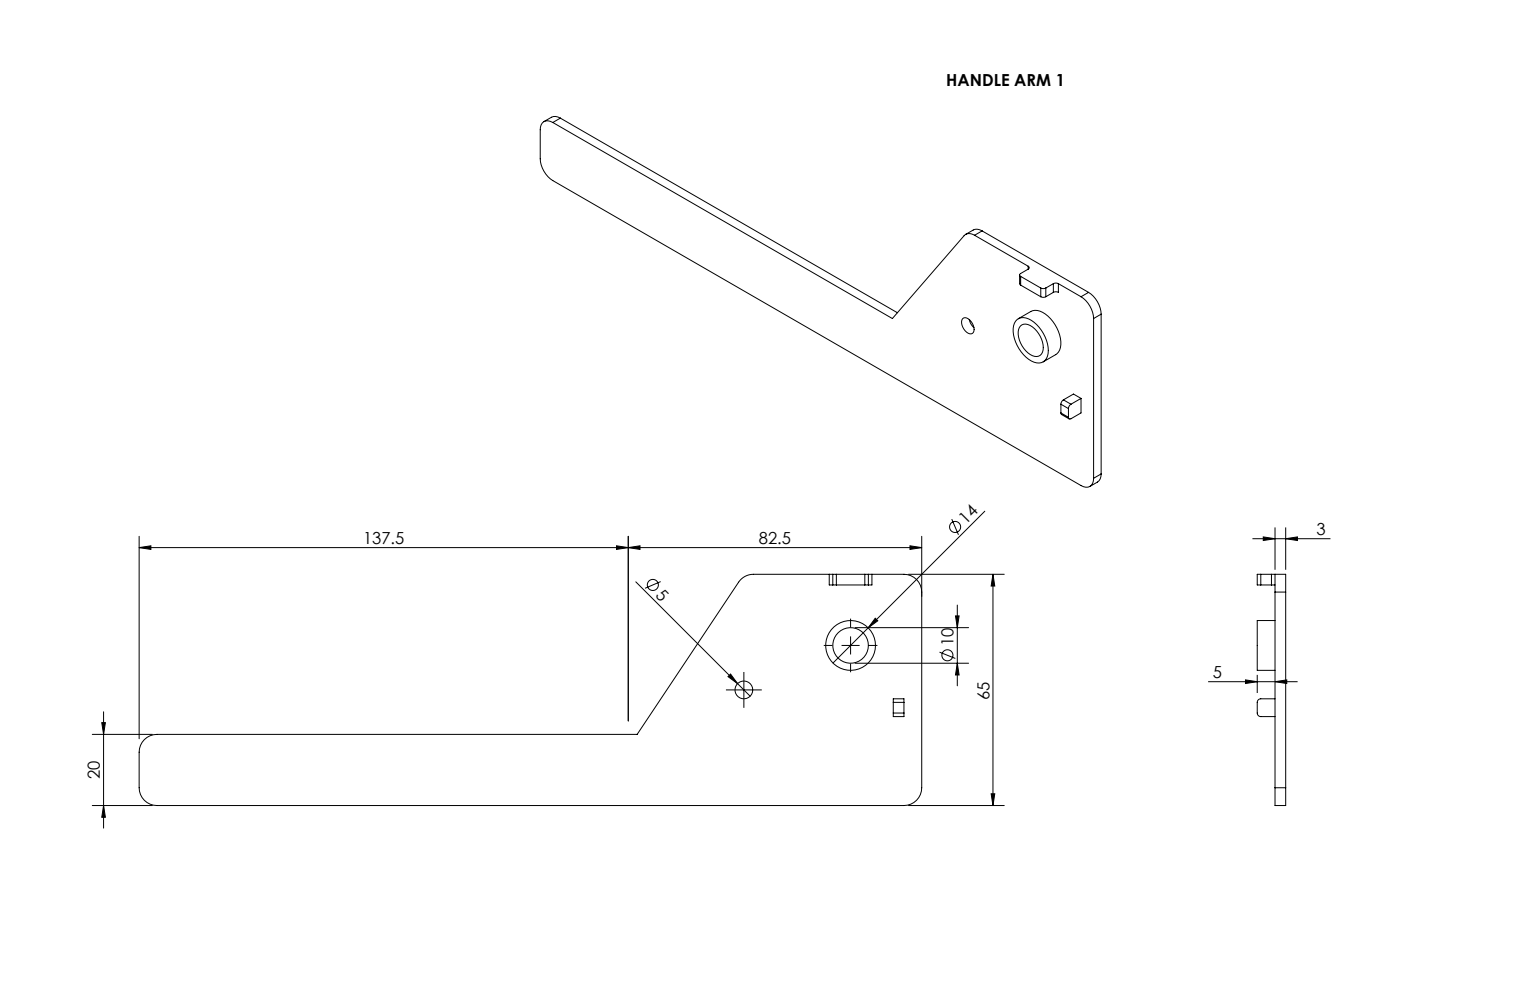
ISO-10303-21;
HEADER;
FILE_DESCRIPTION (('STEP AP214'),
    '1' );
FILE_NAME ('Handle Arm 1.step',
    '2026-09-24T10:15:42',
    ( '' ),
    ( '' ),
    'SwSTEP 2.0',
    'SolidWorks 2026',
    '' );
FILE_SCHEMA (( 'AUTOMOTIVE_DESIGN' ));
ENDSEC;

DATA;
#1=PRODUCT_DEFINITION_CONTEXT ( 'detailed design', #13776, 'design' ) ;
#12=DIRECTION ( 'NONE',  ( -1.000000000000000000, 0.000000000000000000, 0.000000000000000000 ) ) ;
#14=ORIENTED_EDGE ( 'NONE', *, *, #2662, .F. ) ;
#26=FACE_BOUND ( 'NONE', #13698, .T. ) ;
#28=DIRECTION ( 'NONE',  ( 0.000000000000000000, 0.000000000000000000, 1.000000000000000000 ) ) ;
#44=DIRECTION ( 'NONE',  ( -0.000000000000000000, 1.000000000000000000, -0.000000000000000000 ) ) ;
#93=ORIENTED_EDGE ( 'NONE', *, *, #12903, .T. ) ;
#95=CIRCLE ( 'NONE', #1308, 7.000000000000000000 ) ;
#113=ORIENTED_EDGE ( 'NONE', *, *, #10115, .F. ) ;
#155=ORIENTED_EDGE ( 'NONE', *, *, #10739, .F. ) ;
#161=AXIS2_PLACEMENT_3D ( 'NONE', #1843, #5935, #10343 ) ;
#162=CARTESIAN_POINT ( 'NONE',  ( 0.000000000000000000, 0.000000000000000000, 3.000000000000000000 ) ) ;
#198=LINE ( 'NONE', #14619, #1257 ) ;
#221=EDGE_CURVE ( 'NONE', #1746, #4825, #4915, .T. ) ;
#222=CARTESIAN_POINT ( 'NONE',  ( -199.9999999999999716, -40.00000000000003553, 0.000000000000000000 ) ) ;
#235=CARTESIAN_POINT ( 'NONE',  ( -7.000000000000000000, 0.000000000000000000, 3.000000000000000000 ) ) ;
#275=DIRECTION ( 'NONE',  ( -0.000000000000000000, -0.000000000000000000, -1.000000000000000000 ) ) ;
#276=ORIENTED_EDGE ( 'NONE', *, *, #18179, .T. ) ;
#278=ORIENTED_EDGE ( 'NONE', *, *, #5786, .T. ) ;
#313=CYLINDRICAL_SURFACE ( 'NONE', #161, 1.000000000000000000 ) ;
#317=CARTESIAN_POINT ( 'NONE',  ( 12.00000000000000711, -19.99999999999999645, 8.000000000000000000 ) ) ;
#358=AXIS2_PLACEMENT_3D ( 'NONE', #13594, #3263, #9294 ) ;
#369=VERTEX_POINT ( 'NONE', #8341 ) ;
#398=CARTESIAN_POINT ( 'NONE',  ( -59.99999999999997158, -25.00000000000000711, 3.000000000000000000 ) ) ;
#407=ORIENTED_EDGE ( 'NONE', *, *, #468, .F. ) ;
#423=ORIENTED_EDGE ( 'NONE', *, *, #6973, .T. ) ;
#425=ORIENTED_EDGE ( 'NONE', *, *, #1863, .T. ) ;
#453=CARTESIAN_POINT ( 'NONE',  ( 5.000000000000000000, 20.00000000000000000, 7.000000000000000000 ) ) ;
#460=VECTOR ( 'NONE', #9280, 1000.000000000000000 ) ;
#468=EDGE_CURVE ( 'NONE', #16237, #16692, #17037, .T. ) ;
#469=ORIENTED_EDGE ( 'NONE', *, *, #3648, .F. ) ;
#474=AXIS2_PLACEMENT_3D ( 'NONE', #15954, #2942, #11381 ) ;
#490=EDGE_CURVE ( 'NONE', #12958, #6376, #11788, .T. ) ;
#515=PLANE ( 'NONE',  #9065 ) ;
#521=ORIENTED_EDGE ( 'NONE', *, *, #6601, .T. ) ;
#522=EDGE_LOOP ( 'NONE', ( #4200, #469, #9794, #11121 ) ) ;
#530=VECTOR ( 'NONE', #4094, 1000.000000000000000 ) ;
#560=EDGE_CURVE ( 'NONE', #16555, #5753, #17707, .T. ) ;
#570=VERTEX_POINT ( 'NONE', #398 ) ;
#573=EDGE_LOOP ( 'NONE', ( #1318, #5480, #17892, #18760, #5656, #10397, #11984, #9259, #13184, #1949, #6060, #18876, #14646, #9892, #5411 ) ) ;
#585=DIRECTION ( 'NONE',  ( -0.000000000000000000, -0.000000000000000000, -1.000000000000000000 ) ) ;
#586=EDGE_CURVE ( 'NONE', #8358, #2858, #15012, .T. ) ;
#615=CARTESIAN_POINT ( 'NONE',  ( 14.99999999999999289, 20.00000000000000000, 3.000000000000000000 ) ) ;
#626=FILL_AREA_STYLE ('',( #13710 ) ) ;
#635=LINE ( 'NONE', #5205, #2069 ) ;
#648=EDGE_CURVE ( 'NONE', #1182, #5121, #7868, .T. ) ;
#692=CARTESIAN_POINT ( 'NONE',  ( 15.00000000000000711, -19.99999999999999645, 8.000000000000000000 ) ) ;
#704=ORIENTED_EDGE ( 'NONE', *, *, #13489, .F. ) ;
#745=EDGE_LOOP ( 'NONE', ( #12051, #16881, #10808, #1545 ) ) ;
#751=AXIS2_PLACEMENT_3D ( 'NONE', #1811, #13461, #4679 ) ;
#753=DIRECTION ( 'NONE',  ( -2.891205793294679312E-16, 1.000000000000000000, -0.000000000000000000 ) ) ;
#761=FACE_OUTER_BOUND ( 'NONE', #16218, .T. ) ;
#805=LINE ( 'NONE', #12460, #8156 ) ;
#815=DIRECTION ( 'NONE',  ( 0.000000000000000000, 1.000000000000000000, 0.000000000000000000 ) ) ;
#839=EDGE_LOOP ( 'NONE', ( #9618, #4136, #7135, #7088 ) ) ;
#862=LINE ( 'NONE', #2380, #530 ) ;
#864=VECTOR ( 'NONE', #14123, 1000.000000000000000 ) ;
#869=CARTESIAN_POINT ( 'NONE',  ( -31.48433267924924550, 17.77350098112614418, 3.000000000000000000 ) ) ;
#952=AXIS2_PLACEMENT_3D ( 'NONE', #17004, #15642, #4089 ) ;
#963=LINE ( 'NONE', #3481, #18162 ) ;
#964=VECTOR ( 'NONE', #10328, 1000.000000000000000 ) ;
#984=EDGE_CURVE ( 'NONE', #4000, #3723, #9255, .T. ) ;
#1011=ORIENTED_EDGE ( 'NONE', *, *, #18077, .T. ) ;
#1034=CIRCLE ( 'NONE', #6558, 5.000000000000000888 ) ;
#1077=CIRCLE ( 'NONE', #5966, 7.000000000000000000 ) ;
#1089=( GEOMETRIC_REPRESENTATION_CONTEXT ( 3 ) GLOBAL_UNCERTAINTY_ASSIGNED_CONTEXT ( ( #4604 ) ) GLOBAL_UNIT_ASSIGNED_CONTEXT ( ( #12759, #3971, #14471 ) ) REPRESENTATION_CONTEXT ( 'NONE', 'WORKASPACE' ) );
#1111=LINE ( 'NONE', #8383, #16047 ) ;
#1121=AXIS2_PLACEMENT_3D ( 'NONE', #8036, #5424, #9728 ) ;
#1130=CIRCLE ( 'NONE', #17008, 1.000000000000000000 ) ;
#1160=EDGE_CURVE ( 'NONE', #17471, #3540, #11075, .T. ) ;
#1171=UNCERTAINTY_MEASURE_WITH_UNIT (LENGTH_MEASURE( 1.000000000000000082E-05 ), #17826, 'distance_accuracy_value', 'NONE');
#1182=VERTEX_POINT ( 'NONE', #2186 ) ;
#1186=EDGE_CURVE ( 'NONE', #5607, #14673, #5331, .T. ) ;
#1194=DIRECTION ( 'NONE',  ( -0.000000000000000000, -0.000000000000000000, -1.000000000000000000 ) ) ;
#1202=( GEOMETRIC_REPRESENTATION_CONTEXT ( 3 ) GLOBAL_UNCERTAINTY_ASSIGNED_CONTEXT ( ( #1171 ) ) GLOBAL_UNIT_ASSIGNED_CONTEXT ( ( #17826, #3665, #10559 ) ) REPRESENTATION_CONTEXT ( 'NONE', 'WORKASPACE' ) );
#1221=CIRCLE ( 'NONE', #2701, 1.000000000000000000 ) ;
#1224=ADVANCED_FACE ( 'NONE', ( #6855 ), #12955, .F. ) ;
#1226=EDGE_LOOP ( 'NONE', ( #3328, #17393 ) ) ;
#1241=EDGE_CURVE ( 'NONE', #18187, #18838, #13054, .T. ) ;
#1244=DIRECTION ( 'NONE',  ( 0.000000000000000000, 0.000000000000000000, 1.000000000000000000 ) ) ;
#1257=VECTOR ( 'NONE', #4220, 1000.000000000000000 ) ;
#1308=AXIS2_PLACEMENT_3D ( 'NONE', #10783, #18228, #8012 ) ;
#1310=CARTESIAN_POINT ( 'NONE',  ( -194.9999999999999716, -25.00000000000003197, 0.000000000000000000 ) ) ;
#1318=ORIENTED_EDGE ( 'NONE', *, *, #5137, .T. ) ;
#1356=CARTESIAN_POINT ( 'NONE',  ( 0.000000000000000000, 0.000000000000000000, 3.000000000000000000 ) ) ;
#1368=DIRECTION ( 'NONE',  ( 1.000000000000000000, -0.000000000000000000, -0.000000000000000000 ) ) ;
#1385=SURFACE_SIDE_STYLE ('',( #10081 ) ) ;
#1387=LINE ( 'NONE', #17642, #18551 ) ;
#1396=COLOUR_RGB ( '', 0.66274510, 0.83137255, 0.94901961) ;
#1417=AXIS2_PLACEMENT_3D ( 'NONE', #8399, #17095, #15747 ) ;
#1429=ORIENTED_EDGE ( 'NONE', *, *, #9598, .F. ) ;
#1432=CARTESIAN_POINT ( 'NONE',  ( -199.9999999999999716, -25.00000000000003197, 3.000000000000000000 ) ) ;
#1440=CIRCLE ( 'NONE', #17939, 1.000000000000000000 ) ;
#1452=DIRECTION ( 'NONE',  ( 0.000000000000000000, 0.000000000000000000, -1.000000000000000000 ) ) ;
#1503=CARTESIAN_POINT ( 'NONE',  ( 0.000000000000000000, -15.99999999999999645, 7.000000000000000000 ) ) ;
#1544=EDGE_CURVE ( 'NONE', #14463, #9042, #14538, .T. ) ;
#1545=ORIENTED_EDGE ( 'NONE', *, *, #3989, .T. ) ;
#1566=VERTEX_POINT ( 'NONE', #9951 ) ;
#1589=FACE_OUTER_BOUND ( 'NONE', #1862, .T. ) ;
#1600=LINE ( 'NONE', #10200, #6143 ) ;
#1608=ORIENTED_EDGE ( 'NONE', *, *, #6091, .F. ) ;
#1654=VECTOR ( 'NONE', #17324, 1000.000000000000000 ) ;
#1660=ADVANCED_FACE ( 'NONE', ( #11871 ), #4607, .F. ) ;
#1668=AXIS2_PLACEMENT_3D ( 'NONE', #5688, #15832, #14585 ) ;
#1710=EDGE_CURVE ( 'NONE', #9189, #11716, #4983, .T. ) ;
#1719=( GEOMETRIC_REPRESENTATION_CONTEXT ( 3 ) GLOBAL_UNCERTAINTY_ASSIGNED_CONTEXT ( ( #13193 ) ) GLOBAL_UNIT_ASSIGNED_CONTEXT ( ( #14378, #12665, #4064 ) ) REPRESENTATION_CONTEXT ( 'NONE', 'WORKASPACE' ) );
#1721=PLANE ( 'NONE',  #4737 ) ;
#1724=ORIENTED_EDGE ( 'NONE', *, *, #586, .F. ) ;
#1743=DIRECTION ( 'NONE',  ( 1.000000000000000000, 0.000000000000000000, 0.000000000000000000 ) ) ;
#1746=VERTEX_POINT ( 'NONE', #12253 ) ;
#1751=LINE ( 'NONE', #16478, #16323 ) ;
#1759=ORIENTED_EDGE ( 'NONE', *, *, #2129, .F. ) ;
#1811=CARTESIAN_POINT ( 'NONE',  ( -194.9999999999999716, -30.00000000000003197, 3.000000000000000000 ) ) ;
#1828=ORIENTED_EDGE ( 'NONE', *, *, #2662, .T. ) ;
#1843=CARTESIAN_POINT ( 'NONE',  ( -6.000000000000000000, 20.00000000000000000, 4.000000000000000000 ) ) ;
#1862=EDGE_LOOP ( 'NONE', ( #3776, #7335, #13877, #5146 ) ) ;
#1863=EDGE_CURVE ( 'NONE', #16885, #9189, #8144, .T. ) ;
#1870=PLANE ( 'NONE',  #10860 ) ;
#1876=VECTOR ( 'NONE', #4466, 1000.000000000000000 ) ;
#1905=CARTESIAN_POINT ( 'NONE',  ( -5.000000000000000888, 17.00000000000000000, 8.000000000000000000 ) ) ;
#1909=CIRCLE ( 'NONE', #18376, 2.499999999999995115 ) ;
#1920=CARTESIAN_POINT ( 'NONE',  ( -5.000000000000000888, 17.00000000000000000, 8.000000000000000000 ) ) ;
#1949=ORIENTED_EDGE ( 'NONE', *, *, #984, .T. ) ;
#1957=FACE_OUTER_BOUND ( 'NONE', #3513, .T. ) ;
#1961=CARTESIAN_POINT ( 'NONE',  ( 12.00000000000000711, -19.99999999999999645, 3.000000000000000000 ) ) ;
#1984=VECTOR ( 'NONE', #6709, 1000.000000000000000 ) ;
#2030=AXIS2_PLACEMENT_3D ( 'NONE', #15716, #11248, #17249 ) ;
#2033=AXIS2_PLACEMENT_3D ( 'NONE', #8613, #9948, #12 ) ;
#2036=LINE ( 'NONE', #692, #12375 ) ;
#2061=AXIS2_PLACEMENT_3D ( 'NONE', #12590, #2277, #3626 ) ;
#2069=VECTOR ( 'NONE', #815, 1000.000000000000000 ) ;
#2085=CARTESIAN_POINT ( 'NONE',  ( 15.00000000000000711, -15.99999999999999645, 7.000000000000000000 ) ) ;
#2112=ADVANCED_FACE ( 'NONE', ( #18885 ), #7343, .T. ) ;
#2118=ORIENTED_EDGE ( 'NONE', *, *, #9241, .T. ) ;
#2129=EDGE_CURVE ( 'NONE', #18838, #8358, #15102, .T. ) ;
#2130=ADVANCED_FACE ( 'NONE', ( #13153 ), #17459, .T. ) ;
#2142=DIRECTION ( 'NONE',  ( 0.000000000000000000, 0.000000000000000000, -1.000000000000000000 ) ) ;
#2169=LINE ( 'NONE', #16970, #15447 ) ;
#2186=CARTESIAN_POINT ( 'NONE',  ( 5.000000000000000888, 17.00000000000000000, 4.000000000000000000 ) ) ;
#2197=CARTESIAN_POINT ( 'NONE',  ( 0.000000000000000000, 0.000000000000000000, 8.000000000000000000 ) ) ;
#2204=ADVANCED_FACE ( 'NONE', ( #17170 ), #15734, .T. ) ;
#2218=LINE ( 'NONE', #7886, #4396 ) ;
#2224=DIRECTION ( 'NONE',  ( -0.000000000000000000, 1.000000000000000000, -0.000000000000000000 ) ) ;
#2230=ORIENTED_EDGE ( 'NONE', *, *, #8585, .T. ) ;
#2231=CARTESIAN_POINT ( 'NONE',  ( 15.00000000000000711, -19.99999999999999645, 3.000000000000000000 ) ) ;
#2245=AXIS2_PLACEMENT_3D ( 'NONE', #18631, #18546, #11384 ) ;
#2254=ORIENTED_EDGE ( 'NONE', *, *, #16024, .F. ) ;
#2268=DIRECTION ( 'NONE',  ( -1.000000000000000000, -0.000000000000000000, -0.000000000000000000 ) ) ;
#2277=DIRECTION ( 'NONE',  ( 2.891205793294679312E-16, -1.000000000000000000, 0.000000000000000000 ) ) ;
#2380=CARTESIAN_POINT ( 'NONE',  ( -5.000000000000000888, 17.00000000000000000, 8.000000000000000000 ) ) ;
#2388=CARTESIAN_POINT ( 'NONE',  ( -199.9999999999999716, -30.00000000000003197, 3.000000000000000000 ) ) ;
#2390=FACE_OUTER_BOUND ( 'NONE', #11983, .T. ) ;
#2438=EDGE_LOOP ( 'NONE', ( #5584, #5199, #7981, #10841 ) ) ;
#2458=ORIENTED_EDGE ( 'NONE', *, *, #9502, .T. ) ;
#2473=LINE ( 'NONE', #5445, #8530 ) ;
#2522=CARTESIAN_POINT ( 'NONE',  ( -7.000000000000000000, 0.000000000000000000, 8.000000000000000000 ) ) ;
#2549=FACE_OUTER_BOUND ( 'NONE', #3127, .T. ) ;
#2569=ADVANCED_FACE ( 'NONE', ( #3178 ), #13135, .T. ) ;
#2604=VERTEX_POINT ( 'NONE', #13798 ) ;
#2618=DIRECTION ( 'NONE',  ( 0.000000000000000000, 0.000000000000000000, -1.000000000000000000 ) ) ;
#2635=VECTOR ( 'NONE', #275, 1000.000000000000000 ) ;
#2651=CIRCLE ( 'NONE', #16093, 5.000000000000000888 ) ;
#2662=EDGE_CURVE ( 'NONE', #15937, #17471, #13615, .T. ) ;
#2665=DIRECTION ( 'NONE',  ( 0.000000000000000000, 0.000000000000000000, -1.000000000000000000 ) ) ;
#2669=EDGE_LOOP ( 'NONE', ( #14305, #3774, #4650, #17336 ) ) ;
#2680=EDGE_CURVE ( 'NONE', #14205, #3723, #805, .T. ) ;
#2701=AXIS2_PLACEMENT_3D ( 'NONE', #16647, #16830, #5259 ) ;
#2725=DIRECTION ( 'NONE',  ( -0.000000000000000000, 0.000000000000000000, 1.000000000000000000 ) ) ;
#2732=LINE ( 'NONE', #12968, #864 ) ;
#2802=ADVANCED_FACE ( 'NONE', ( #12634 ), #18845, .F. ) ;
#2806=AXIS2_PLACEMENT_3D ( 'NONE', #2197, #12505, #6691 ) ;
#2812=DIRECTION ( 'NONE',  ( -0.000000000000000000, -0.000000000000000000, -1.000000000000000000 ) ) ;
#2824=ORIENTED_EDGE ( 'NONE', *, *, #7779, .T. ) ;
#2827=EDGE_CURVE ( 'NONE', #12087, #16455, #10055, .T. ) ;
#2850=DIRECTION ( 'NONE',  ( -0.000000000000000000, -0.000000000000000000, -1.000000000000000000 ) ) ;
#2858=VERTEX_POINT ( 'NONE', #14165 ) ;
#2878=EDGE_LOOP ( 'NONE', ( #15032, #425, #13147, #2999 ) ) ;
#2942=DIRECTION ( 'NONE',  ( 0.000000000000000000, 0.000000000000000000, 1.000000000000000000 ) ) ;
#2962=CARTESIAN_POINT ( 'NONE',  ( -31.48433267924924550, 17.77350098112614418, 3.000000000000000000 ) ) ;
#2999=ORIENTED_EDGE ( 'NONE', *, *, #18071, .F. ) ;
#3009=CARTESIAN_POINT ( 'NONE',  ( 19.99999999999999645, 20.00000000000000000, 0.000000000000000000 ) ) ;
#3045=EDGE_CURVE ( 'NONE', #9189, #8319, #3244, .T. ) ;
#3067=ORIENTED_EDGE ( 'NONE', *, *, #221, .T. ) ;
#3096=ORIENTED_EDGE ( 'NONE', *, *, #8885, .F. ) ;
#3097=ADVANCED_FACE ( 'NONE', ( #16726 ), #15371, .F. ) ;
#3101=FACE_BOUND ( 'NONE', #522, .T. ) ;
#3127=EDGE_LOOP ( 'NONE', ( #13679, #11435, #11316, #6059 ) ) ;
#3136=VERTEX_POINT ( 'NONE', #5333 ) ;
#3138=DIRECTION ( 'NONE',  ( -0.000000000000000000, -0.000000000000000000, 1.000000000000000000 ) ) ;
#3149=CARTESIAN_POINT ( 'NONE',  ( -30.00000000000000711, 20.00000000000000000, 3.000000000000000000 ) ) ;
#3167=DIRECTION ( 'NONE',  ( 1.000000000000000000, 0.000000000000000000, 0.000000000000000000 ) ) ;
#3178=FACE_OUTER_BOUND ( 'NONE', #16382, .T. ) ;
#3217=ORIENTED_EDGE ( 'NONE', *, *, #6850, .F. ) ;
#3232=DIRECTION ( 'NONE',  ( -1.000000000000000000, 0.000000000000000000, 0.000000000000000000 ) ) ;
#3244=CIRCLE ( 'NONE', #1121, 5.000000000000000888 ) ;
#3263=DIRECTION ( 'NONE',  ( 0.000000000000000000, 0.000000000000000000, -1.000000000000000000 ) ) ;
#3268=CARTESIAN_POINT ( 'NONE',  ( -5.000000000000000888, 17.00000000000000000, 3.000000000000000000 ) ) ;
#3281=AXIS2_PLACEMENT_3D ( 'NONE', #9441, #2618, #15718 ) ;
#3282=CARTESIAN_POINT ( 'NONE',  ( 12.00000000000000711, -18.99999999999999645, 7.000000000000000000 ) ) ;
#3287=CARTESIAN_POINT ( 'NONE',  ( -27.50000000000000711, -12.50000000000000178, 3.000000000000000000 ) ) ;
#3298=ORIENTED_EDGE ( 'NONE', *, *, #8499, .F. ) ;
#3328=ORIENTED_EDGE ( 'NONE', *, *, #7688, .T. ) ;
#3361=DIRECTION ( 'NONE',  ( -1.000000000000000000, 0.000000000000000000, 0.000000000000000000 ) ) ;
#3362=CARTESIAN_POINT ( 'NONE',  ( -27.32408120756002035, 15.00000000000000000, 3.000000000000000000 ) ) ;
#3368=DIRECTION ( 'NONE',  ( 2.891205793294679312E-16, -1.000000000000000000, 0.000000000000000000 ) ) ;
#3423=LINE ( 'NONE', #13460, #18761 ) ;
#3436=EDGE_CURVE ( 'NONE', #6376, #6155, #7941, .T. ) ;
#3438=EDGE_CURVE ( 'NONE', #14673, #9334, #16720, .T. ) ;
#3461=DIRECTION ( 'NONE',  ( -1.577021341797097560E-16, 1.000000000000000000, 0.000000000000000000 ) ) ;
#3462=ORIENTED_EDGE ( 'NONE', *, *, #15222, .T. ) ;
#3481=CARTESIAN_POINT ( 'NONE',  ( -59.99999999999997158, -25.00000000000000711, 3.000000000000000000 ) ) ;
#3506=AXIS2_PLACEMENT_3D ( 'NONE', #12271, #6728, #18193 ) ;
#3513=EDGE_LOOP ( 'NONE', ( #16153, #14510, #9894, #11746 ) ) ;
#3517=CIRCLE ( 'NONE', #9325, 1.000000000000000000 ) ;
#3527=ORIENTED_EDGE ( 'NONE', *, *, #15997, .T. ) ;
#3532=CYLINDRICAL_SURFACE ( 'NONE', #9933, 5.000000000000000888 ) ;
#3540=VERTEX_POINT ( 'NONE', #1961 ) ;
#3556=CARTESIAN_POINT ( 'NONE',  ( -59.99999999999997158, -25.00000000000000711, 3.000000000000000000 ) ) ;
#3557=DIRECTION ( 'NONE',  ( 0.000000000000000000, -1.000000000000000000, 0.000000000000000000 ) ) ;
#3558=FACE_OUTER_BOUND ( 'NONE', #13481, .T. ) ;
#3576=VECTOR ( 'NONE', #1452, 1000.000000000000000 ) ;
#3589=MANIFOLD_SOLID_BREP ( 'Extrude-Thin1', #12430 ) ;
#3600=ORIENTED_EDGE ( 'NONE', *, *, #15222, .F. ) ;
#3606=CYLINDRICAL_SURFACE ( 'NONE', #3281, 5.000000000000000888 ) ;
#3608=CARTESIAN_POINT ( 'NONE',  ( 4.000000000000000000, 17.00000000000000000, 8.000000000000000000 ) ) ;
#3620=CARTESIAN_POINT ( 'NONE',  ( 4.000000000000000000, 20.00000000000000000, 8.000000000000000000 ) ) ;
#3626=DIRECTION ( 'NONE',  ( 1.000000000000000000, 0.000000000000000000, 0.000000000000000000 ) ) ;
#3627=FACE_OUTER_BOUND ( 'NONE', #18651, .T. ) ;
#3648=EDGE_CURVE ( 'NONE', #3540, #11936, #5548, .T. ) ;
#3665=( NAMED_UNIT ( * ) PLANE_ANGLE_UNIT ( ) SI_UNIT ( $, .RADIAN. ) );
#3718=DIRECTION ( 'NONE',  ( -0.000000000000000000, -0.000000000000000000, 1.000000000000000000 ) ) ;
#3723=VERTEX_POINT ( 'NONE', #10050 ) ;
#3727=ADVANCED_FACE ( 'NONE', ( #5639 ), #16169, .F. ) ;
#3748=ORIENTED_EDGE ( 'NONE', *, *, #3438, .F. ) ;
#3774=ORIENTED_EDGE ( 'NONE', *, *, #468, .T. ) ;
#3776=ORIENTED_EDGE ( 'NONE', *, *, #16532, .F. ) ;
#3783=LINE ( 'NONE', #8195, #16586 ) ;
#3813=EDGE_LOOP ( 'NONE', ( #407, #14321, #14508, #13808 ) ) ;
#3844=STYLED_ITEM ( 'NONE', ( #14296 ), #10845 ) ;
#3848=ORIENTED_EDGE ( 'NONE', *, *, #6525, .F. ) ;
#3889=ORIENTED_EDGE ( 'NONE', *, *, #5137, .F. ) ;
#3960=LINE ( 'NONE', #16776, #13659 ) ;
#3971=( NAMED_UNIT ( * ) PLANE_ANGLE_UNIT ( ) SI_UNIT ( $, .RADIAN. ) );
#3989=EDGE_CURVE ( 'NONE', #369, #14405, #2473, .T. ) ;
#4000=VERTEX_POINT ( 'NONE', #2388 ) ;
#4021=DIRECTION ( 'NONE',  ( -1.000000000000000000, 0.000000000000000000, -0.000000000000000000 ) ) ;
#4064=( NAMED_UNIT ( * ) SI_UNIT ( $, .STERADIAN. ) SOLID_ANGLE_UNIT ( ) );
#4074=ADVANCED_FACE ( 'NONE', ( #17288 ), #5618, .F. ) ;
#4089=DIRECTION ( 'NONE',  ( 1.601283208593975514E-16, -1.000000000000000000, 0.000000000000000000 ) ) ;
#4094=DIRECTION ( 'NONE',  ( -0.000000000000000000, -0.000000000000000000, -1.000000000000000000 ) ) ;
#4111=DIRECTION ( 'NONE',  ( 0.000000000000000000, 0.000000000000000000, 1.000000000000000000 ) ) ;
#4119=CARTESIAN_POINT ( 'NONE',  ( 0.000000000000000000, 0.000000000000000000, 0.000000000000000000 ) ) ;
#4121=ORIENTED_EDGE ( 'NONE', *, *, #8585, .F. ) ;
#4131=DIRECTION ( 'NONE',  ( 2.891205793294679312E-16, -1.000000000000000000, 0.000000000000000000 ) ) ;
#4134=DIRECTION ( 'NONE',  ( -0.000000000000000000, -0.000000000000000000, -1.000000000000000000 ) ) ;
#4136=ORIENTED_EDGE ( 'NONE', *, *, #2680, .T. ) ;
#4164=SHAPE_REPRESENTATION_RELATIONSHIP ( 'NONE' , 'NONE' ,  #9113, #10845 ) ;
#4198=VECTOR ( 'NONE', #17813, 1000.000000000000000 ) ;
#4200=ORIENTED_EDGE ( 'NONE', *, *, #5975, .F. ) ;
#4220=DIRECTION ( 'NONE',  ( 2.891205793294679312E-16, 1.000000000000000000, -0.000000000000000000 ) ) ;
#4279=LINE ( 'NONE', #3009, #1876 ) ;
#4323=AXIS2_PLACEMENT_3D ( 'NONE', #16567, #9108, #3361 ) ;
#4374=CARTESIAN_POINT ( 'NONE',  ( 15.00000000000000711, -14.99999999999999645, 3.000000000000000000 ) ) ;
#4396=VECTOR ( 'NONE', #6434, 1000.000000000000000 ) ;
#4409=CARTESIAN_POINT ( 'NONE',  ( 5.000000000000000000, 20.00000000000000000, 8.000000000000000000 ) ) ;
#4420=CARTESIAN_POINT ( 'NONE',  ( 5.000000000000000000, 20.00000000000000000, 4.000000000000000000 ) ) ;
#4421=DIRECTION ( 'NONE',  ( 0.000000000000000000, 0.000000000000000000, -1.000000000000000000 ) ) ;
#4440=CIRCLE ( 'NONE', #9931, 1.000000000000000000 ) ;
#4451=ORIENTED_EDGE ( 'NONE', *, *, #3045, .T. ) ;
#4460=FACE_OUTER_BOUND ( 'NONE', #573, .T. ) ;
#4466=DIRECTION ( 'NONE',  ( -1.601283208593975514E-16, 1.000000000000000000, -0.000000000000000000 ) ) ;
#4471=LINE ( 'NONE', #5891, #18430 ) ;
#4482=CIRCLE ( 'NONE', #6924, 5.000000000000004441 ) ;
#4505=CARTESIAN_POINT ( 'NONE',  ( -27.32408120756002035, 20.00000000000000000, 3.000000000000000000 ) ) ;
#4509=DIRECTION ( 'NONE',  ( 1.000000000000000000, 0.000000000000000000, 0.000000000000000000 ) ) ;
#4519=DIRECTION ( 'NONE',  ( 0.000000000000000000, 0.000000000000000000, 1.000000000000000000 ) ) ;
#4587=VERTEX_POINT ( 'NONE', #453 ) ;
#4598=CYLINDRICAL_SURFACE ( 'NONE', #9372, 5.000000000000000000 ) ;
#4604=UNCERTAINTY_MEASURE_WITH_UNIT (LENGTH_MEASURE( 1.000000000000000082E-05 ), #12759, 'distance_accuracy_value', 'NONE');
#4607=PLANE ( 'NONE',  #18519 ) ;
#4612=VECTOR ( 'NONE', #7351, 1000.000000000000000 ) ;
#4626=AXIS2_PLACEMENT_3D ( 'NONE', #13967, #1244, #16931 ) ;
#4628=ORIENTED_EDGE ( 'NONE', *, *, #8885, .T. ) ;
#4650=ORIENTED_EDGE ( 'NONE', *, *, #18545, .T. ) ;
#4651=ORIENTED_EDGE ( 'NONE', *, *, #490, .F. ) ;
#4677=CARTESIAN_POINT ( 'NONE',  ( -199.9999999999999716, -25.00000000000003197, 3.000000000000000000 ) ) ;
#4679=DIRECTION ( 'NONE',  ( -1.000000000000000000, 0.000000000000000000, 0.000000000000000000 ) ) ;
#4737=AXIS2_PLACEMENT_3D ( 'NONE', #1920, #10710, #7371 ) ;
#4764=AXIS2_PLACEMENT_3D ( 'NONE', #17152, #1194, #18673 ) ;
#4788=EDGE_LOOP ( 'NONE', ( #12454, #11557 ) ) ;
#4796=DIRECTION ( 'NONE',  ( -2.891205793294679312E-16, 1.000000000000000000, 0.000000000000000000 ) ) ;
#4801=DIRECTION ( 'NONE',  ( 0.5547001962252284812, 0.8320502943378440541, 0.000000000000000000 ) ) ;
#4825=VERTEX_POINT ( 'NONE', #14330 ) ;
#4903=LINE ( 'NONE', #3556, #8350 ) ;
#4910=ORIENTED_EDGE ( 'NONE', *, *, #1863, .F. ) ;
#4915=LINE ( 'NONE', #11888, #5141 ) ;
#4942=EDGE_CURVE ( 'NONE', #18779, #4000, #5017, .T. ) ;
#4983=LINE ( 'NONE', #10819, #8456 ) ;
#5004=EDGE_CURVE ( 'NONE', #16605, #7666, #18852, .T. ) ;
#5017=CIRCLE ( 'NONE', #751, 5.000000000000004441 ) ;
#5024=EDGE_LOOP ( 'NONE', ( #18369, #18554, #12205, #13177 ) ) ;
#5058=CARTESIAN_POINT ( 'NONE',  ( -27.32408120756002035, 15.00000000000000000, 3.000000000000000000 ) ) ;
#5059=CARTESIAN_POINT ( 'NONE',  ( -7.000000000000000000, 0.000000000000000000, 8.000000000000000000 ) ) ;
#5062=AXIS2_PLACEMENT_3D ( 'NONE', #18421, #585, #5149 ) ;
#5121=VERTEX_POINT ( 'NONE', #4420 ) ;
#5135=ORIENTED_EDGE ( 'NONE', *, *, #12903, .F. ) ;
#5137=EDGE_CURVE ( 'NONE', #6376, #6854, #1751, .T. ) ;
#5141=VECTOR ( 'NONE', #13606, 1000.000000000000000 ) ;
#5146=ORIENTED_EDGE ( 'NONE', *, *, #3989, .F. ) ;
#5149=DIRECTION ( 'NONE',  ( -1.000000000000000000, 0.000000000000000000, 0.000000000000000000 ) ) ;
#5158=EDGE_CURVE ( 'NONE', #5753, #16885, #1034, .T. ) ;
#5175=FACE_OUTER_BOUND ( 'NONE', #12880, .T. ) ;
#5199=ORIENTED_EDGE ( 'NONE', *, *, #9706, .T. ) ;
#5205=CARTESIAN_POINT ( 'NONE',  ( 15.00000000000000711, -19.99999999999999645, 3.000000000000000000 ) ) ;
#5211=EDGE_CURVE ( 'NONE', #9296, #3540, #2218, .T. ) ;
#5220=CARTESIAN_POINT ( 'NONE',  ( -194.9999999999999716, -25.00000000000003197, 3.000000000000000000 ) ) ;
#5239=ADVANCED_FACE ( 'NONE', ( #3558 ), #515, .F. ) ;
#5249=ORIENTED_EDGE ( 'NONE', *, *, #648, .T. ) ;
#5259=DIRECTION ( 'NONE',  ( 0.000000000000000000, 0.000000000000000000, -1.000000000000000000 ) ) ;
#5265=CARTESIAN_POINT ( 'NONE',  ( -59.99999999999997158, -25.00000000000000711, 0.000000000000000000 ) ) ;
#5275=VERTEX_POINT ( 'NONE', #16932 ) ;
#5320=CARTESIAN_POINT ( 'NONE',  ( 12.00000000000000711, -19.99999999999999645, 8.000000000000000000 ) ) ;
#5331=CIRCLE ( 'NONE', #9601, 1.000000000000000000 ) ;
#5333=CARTESIAN_POINT ( 'NONE',  ( 12.00000000000000711, -15.99999999999999645, 8.000000000000000000 ) ) ;
#5411=ORIENTED_EDGE ( 'NONE', *, *, #490, .T. ) ;
#5412=ORIENTED_EDGE ( 'NONE', *, *, #12668, .T. ) ;
#5424=DIRECTION ( 'NONE',  ( 0.000000000000000000, 0.000000000000000000, -1.000000000000000000 ) ) ;
#5445=CARTESIAN_POINT ( 'NONE',  ( -4.000000000000000888, 17.00000000000000000, 8.000000000000000000 ) ) ;
#5448=CARTESIAN_POINT ( 'NONE',  ( 15.00000000000000711, -18.99999999999999645, 8.000000000000000000 ) ) ;
#5480=ORIENTED_EDGE ( 'NONE', *, *, #12072, .T. ) ;
#5511=ADVANCED_FACE ( 'NONE', ( #8799 ), #4598, .F. ) ;
#5548=LINE ( 'NONE', #2231, #17998 ) ;
#5564=VERTEX_POINT ( 'NONE', #7958 ) ;
#5584=ORIENTED_EDGE ( 'NONE', *, *, #7779, .F. ) ;
#5588=CARTESIAN_POINT ( 'NONE',  ( 15.00000000000000711, -45.00000000000000000, 3.000000000000000000 ) ) ;
#5607=VERTEX_POINT ( 'NONE', #12426 ) ;
#5618=PLANE ( 'NONE',  #10361 ) ;
#5637=ORIENTED_EDGE ( 'NONE', *, *, #9706, .F. ) ;
#5639=FACE_OUTER_BOUND ( 'NONE', #6609, .T. ) ;
#5656=ORIENTED_EDGE ( 'NONE', *, *, #560, .T. ) ;
#5663=CIRCLE ( 'NONE', #12999, 1.000000000000000000 ) ;
#5674=ORIENTED_EDGE ( 'NONE', *, *, #12977, .T. ) ;
#5682=CARTESIAN_POINT ( 'NONE',  ( 4.000000000000000888, 17.00000000000000000, 7.000000000000000000 ) ) ;
#5688=CARTESIAN_POINT ( 'NONE',  ( 15.00000000000000711, -39.99999999999999289, 3.000000000000000000 ) ) ;
#5699=EDGE_CURVE ( 'NONE', #11329, #12087, #13643, .T. ) ;
#5746=EDGE_CURVE ( 'NONE', #3723, #14463, #4482, .T. ) ;
#5753=VERTEX_POINT ( 'NONE', #14042 ) ;
#5779=ADVANCED_FACE ( 'NONE', ( #2549 ), #10280, .T. ) ;
#5786=EDGE_CURVE ( 'NONE', #16287, #13879, #14861, .T. ) ;
#5839=CIRCLE ( 'NONE', #15930, 5.000000000000000000 ) ;
#5844=PLANE ( 'NONE',  #15783 ) ;
#5853=AXIS2_PLACEMENT_3D ( 'NONE', #10071, #2268, #6584 ) ;
#5868=LINE ( 'NONE', #11809, #13541 ) ;
#5887=CARTESIAN_POINT ( 'NONE',  ( 5.000000000000000888, 17.00000000000000000, 8.000000000000000000 ) ) ;
#5891=CARTESIAN_POINT ( 'NONE',  ( 5.000000000000000000, 20.00000000000000000, 8.000000000000000000 ) ) ;
#5935=DIRECTION ( 'NONE',  ( 2.891205793294679312E-16, 1.000000000000000000, 0.000000000000000000 ) ) ;
#5955=CYLINDRICAL_SURFACE ( 'NONE', #6494, 2.499999999999992006 ) ;
#5966=AXIS2_PLACEMENT_3D ( 'NONE', #8128, #3718, #13940 ) ;
#5973=EDGE_CURVE ( 'NONE', #9042, #18187, #3960, .T. ) ;
#5975=EDGE_CURVE ( 'NONE', #11936, #14717, #635, .T. ) ;
#5982=ORIENTED_EDGE ( 'NONE', *, *, #3436, .T. ) ;
#5992=LINE ( 'NONE', #5887, #7683 ) ;
#6010=VECTOR ( 'NONE', #10977, 1000.000000000000000 ) ;
#6046=FACE_OUTER_BOUND ( 'NONE', #5024, .T. ) ;
#6055=ORIENTED_EDGE ( 'NONE', *, *, #6489, .F. ) ;
#6059=ORIENTED_EDGE ( 'NONE', *, *, #1544, .F. ) ;
#6060=ORIENTED_EDGE ( 'NONE', *, *, #5746, .T. ) ;
#6083=ORIENTED_EDGE ( 'NONE', *, *, #14312, .T. ) ;
#6091=EDGE_CURVE ( 'NONE', #2604, #15937, #1130, .T. ) ;
#6110=LINE ( 'NONE', #1905, #8606 ) ;
#6122=DIRECTION ( 'NONE',  ( 0.000000000000000000, 0.000000000000000000, -1.000000000000000000 ) ) ;
#6143=VECTOR ( 'NONE', #8776, 1000.000000000000000 ) ;
#6155=VERTEX_POINT ( 'NONE', #14647 ) ;
#6156=VECTOR ( 'NONE', #3557, 1000.000000000000000 ) ;
#6160=DIRECTION ( 'NONE',  ( -1.000000000000000000, 0.000000000000000000, 0.000000000000000000 ) ) ;
#6164=DIRECTION ( 'NONE',  ( 1.000000000000000000, 0.000000000000000000, -0.000000000000000000 ) ) ;
#6203=CARTESIAN_POINT ( 'NONE',  ( -27.32408120756002035, 20.00000000000000000, 0.000000000000000000 ) ) ;
#6221=CARTESIAN_POINT ( 'NONE',  ( 15.00000000000000711, -19.99999999999999645, 7.000000000000000000 ) ) ;
#6225=DIRECTION ( 'NONE',  ( 0.000000000000000000, 0.000000000000000000, 1.000000000000000000 ) ) ;
#6258=AXIS2_PLACEMENT_3D ( 'NONE', #14109, #6959, #11440 ) ;
#6262=DIRECTION ( 'NONE',  ( 0.000000000000000000, -1.000000000000000000, 0.000000000000000000 ) ) ;
#6268=AXIS2_PLACEMENT_3D ( 'NONE', #3282, #17929, #7804 ) ;
#6301=VERTEX_POINT ( 'NONE', #16572 ) ;
#6325=VECTOR ( 'NONE', #3167, 1000.000000000000000 ) ;
#6376=VERTEX_POINT ( 'NONE', #615 ) ;
#6423=ORIENTED_EDGE ( 'NONE', *, *, #15997, .F. ) ;
#6433=CYLINDRICAL_SURFACE ( 'NONE', #358, 5.000000000000000888 ) ;
#6434=DIRECTION ( 'NONE',  ( -0.000000000000000000, -1.000000000000000000, -0.000000000000000000 ) ) ;
#6442=ORIENTED_EDGE ( 'NONE', *, *, #5211, .T. ) ;
#6450=SURFACE_SIDE_STYLE ('',( #12363 ) ) ;
#6453=DIRECTION ( 'NONE',  ( -1.000000000000000000, 0.000000000000000000, -0.000000000000000000 ) ) ;
#6479=FACE_OUTER_BOUND ( 'NONE', #10978, .T. ) ;
#6489=EDGE_CURVE ( 'NONE', #4587, #5607, #9756, .T. ) ;
#6494=AXIS2_PLACEMENT_3D ( 'NONE', #17822, #9122, #8918 ) ;
#6525=EDGE_CURVE ( 'NONE', #16455, #1566, #1909, .T. ) ;
#6529=CARTESIAN_POINT ( 'NONE',  ( -199.9999999999999716, -25.00000000000003197, 0.000000000000000000 ) ) ;
#6540=PLANE ( 'NONE',  #3506 ) ;
#6558=AXIS2_PLACEMENT_3D ( 'NONE', #3362, #10254, #16086 ) ;
#6579=ORIENTED_EDGE ( 'NONE', *, *, #18312, .F. ) ;
#6584=DIRECTION ( 'NONE',  ( 0.000000000000000000, 0.000000000000000000, -1.000000000000000000 ) ) ;
#6586=LINE ( 'NONE', #7747, #11140 ) ;
#6601=EDGE_CURVE ( 'NONE', #11517, #13667, #5839, .T. ) ;
#6609=EDGE_LOOP ( 'NONE', ( #5674, #5249, #155, #17840 ) ) ;
#6636=AXIS2_PLACEMENT_3D ( 'NONE', #14126, #12696, #18527 ) ;
#6639=CIRCLE ( 'NONE', #7552, 1.000000000000000000 ) ;
#6673=ORIENTED_EDGE ( 'NONE', *, *, #9598, .T. ) ;
#6691=DIRECTION ( 'NONE',  ( -1.000000000000000000, 0.000000000000000000, 0.000000000000000000 ) ) ;
#6698=DIRECTION ( 'NONE',  ( -0.000000000000000000, -0.000000000000000000, 1.000000000000000000 ) ) ;
#6709=DIRECTION ( 'NONE',  ( 0.000000000000000000, 0.000000000000000000, -1.000000000000000000 ) ) ;
#6710=VECTOR ( 'NONE', #10899, 1000.000000000000000 ) ;
#6728=DIRECTION ( 'NONE',  ( 0.000000000000000000, -1.000000000000000000, 0.000000000000000000 ) ) ;
#6771=VECTOR ( 'NONE', #3138, 1000.000000000000000 ) ;
#6798=DIRECTION ( 'NONE',  ( -0.000000000000000000, -0.000000000000000000, -1.000000000000000000 ) ) ;
#6803=DIRECTION ( 'NONE',  ( 0.000000000000000000, 0.000000000000000000, -1.000000000000000000 ) ) ;
#6850=EDGE_CURVE ( 'NONE', #14405, #14673, #6110, .T. ) ;
#6854=VERTEX_POINT ( 'NONE', #10607 ) ;
#6855=FACE_OUTER_BOUND ( 'NONE', #18318, .T. ) ;
#6864=VECTOR ( 'NONE', #15087, 1000.000000000000000 ) ;
#6873=DIRECTION ( 'NONE',  ( 0.000000000000000000, 0.000000000000000000, -1.000000000000000000 ) ) ;
#6902=VECTOR ( 'NONE', #4796, 1000.000000000000000 ) ;
#6916=ORIENTED_EDGE ( 'NONE', *, *, #12795, .T. ) ;
#6924=AXIS2_PLACEMENT_3D ( 'NONE', #12786, #14669, #11715 ) ;
#6944=DIRECTION ( 'NONE',  ( 0.000000000000000000, 0.000000000000000000, 1.000000000000000000 ) ) ;
#6959=DIRECTION ( 'NONE',  ( -1.000000000000000000, 0.000000000000000000, 0.000000000000000000 ) ) ;
#6964=VERTEX_POINT ( 'NONE', #8118 ) ;
#6973=EDGE_CURVE ( 'NONE', #3136, #1746, #8919, .T. ) ;
#6979=LINE ( 'NONE', #15292, #8149 ) ;
#6982=ORIENTED_EDGE ( 'NONE', *, *, #12536, .T. ) ;
#6991=PLANE ( 'NONE',  #8694 ) ;
#7074=ORIENTED_EDGE ( 'NONE', *, *, #18112, .T. ) ;
#7088=ORIENTED_EDGE ( 'NONE', *, *, #8814, .T. ) ;
#7101=EDGE_LOOP ( 'NONE', ( #7074, #521 ) ) ;
#7107=CARTESIAN_POINT ( 'NONE',  ( 6.000000000000000888, 17.00000000000000000, 4.000000000000000000 ) ) ;
#7133=VERTEX_POINT ( 'NONE', #235 ) ;
#7135=ORIENTED_EDGE ( 'NONE', *, *, #984, .F. ) ;
#7159=EDGE_LOOP ( 'NONE', ( #15750, #6055, #113, #3748 ) ) ;
#7184=CARTESIAN_POINT ( 'NONE',  ( 19.99999999999999645, 15.00000000000000000, 3.000000000000000000 ) ) ;
#7200=EDGE_CURVE ( 'NONE', #7133, #16692, #18087, .T. ) ;
#7201=ADVANCED_FACE ( 'NONE', ( #13508 ), #5955, .F. ) ;
#7222=AXIS2_PLACEMENT_3D ( 'NONE', #2085, #8740, #14289 ) ;
#7235=VECTOR ( 'NONE', #6453, 1000.000000000000000 ) ;
#7241=DIRECTION ( 'NONE',  ( 2.602085213965210642E-15, 0.000000000000000000, 1.000000000000000000 ) ) ;
#7242=FACE_BOUND ( 'NONE', #13550, .T. ) ;
#7243=CYLINDRICAL_SURFACE ( 'NONE', #14834, 1.000000000000000000 ) ;
#7250=FACE_OUTER_BOUND ( 'NONE', #13130, .T. ) ;
#7272=DIRECTION ( 'NONE',  ( 1.000000000000000000, 0.000000000000000000, -0.000000000000000000 ) ) ;
#7284=ADVANCED_FACE ( 'NONE', ( #16491 ), #6540, .F. ) ;
#7289=DIRECTION ( 'NONE',  ( -0.000000000000000000, -0.000000000000000000, -1.000000000000000000 ) ) ;
#7312=ORIENTED_EDGE ( 'NONE', *, *, #2827, .T. ) ;
#7324=CARTESIAN_POINT ( 'NONE',  ( 5.000000000000000000, 6.123233995736766282E-16, 8.000000000000000000 ) ) ;
#7326=ADVANCED_FACE ( 'NONE', ( #1957 ), #7794, .F. ) ;
#7335=ORIENTED_EDGE ( 'NONE', *, *, #9135, .F. ) ;
#7341=DIRECTION ( 'NONE',  ( 2.891205793294679312E-16, 1.000000000000000000, 0.000000000000000000 ) ) ;
#7343=PLANE ( 'NONE',  #10840 ) ;
#7351=DIRECTION ( 'NONE',  ( -1.000000000000000000, 0.000000000000000000, 0.000000000000000000 ) ) ;
#7371=DIRECTION ( 'NONE',  ( 0.000000000000000000, -0.000000000000000000, 1.000000000000000000 ) ) ;
#7375=ORIENTED_EDGE ( 'NONE', *, *, #18179, .F. ) ;
#7388=CARTESIAN_POINT ( 'NONE',  ( 0.000000000000000000, 0.000000000000000000, 8.000000000000000000 ) ) ;
#7422=DIRECTION ( 'NONE',  ( 2.891205793294679312E-16, -1.000000000000000000, -0.000000000000000000 ) ) ;
#7432=PLANE ( 'NONE',  #16650 ) ;
#7458=CARTESIAN_POINT ( 'NONE',  ( -5.000000000000000000, 20.00000000000000000, 4.000000000000000000 ) ) ;
#7477=CARTESIAN_POINT ( 'NONE',  ( -30.00000000000000711, 20.00000000000000000, 3.000000000000000000 ) ) ;
#7505=DIRECTION ( 'NONE',  ( -0.000000000000000000, -0.000000000000000000, 1.000000000000000000 ) ) ;
#7552=AXIS2_PLACEMENT_3D ( 'NONE', #7107, #9593, #11323 ) ;
#7594=CARTESIAN_POINT ( 'NONE',  ( 5.000000000000000000, 6.123233995736766282E-16, 0.000000000000000000 ) ) ;
#7595=DIRECTION ( 'NONE',  ( -0.000000000000000000, -1.000000000000000000, -0.000000000000000000 ) ) ;
#7598=FACE_OUTER_BOUND ( 'NONE', #8758, .T. ) ;
#7646=CARTESIAN_POINT ( 'NONE',  ( 12.00000000000000711, -14.99999999999999645, 8.000000000000000000 ) ) ;
#7656=CARTESIAN_POINT ( 'NONE',  ( 20.00000000000000711, -39.99999999999999289, 3.000000000000000000 ) ) ;
#7666=VERTEX_POINT ( 'NONE', #7458 ) ;
#7683=VECTOR ( 'NONE', #10102, 1000.000000000000000 ) ;
#7688=EDGE_CURVE ( 'NONE', #1566, #16455, #13884, .T. ) ;
#7704=SURFACE_STYLE_USAGE ( .BOTH. , #6450 ) ;
#7747=CARTESIAN_POINT ( 'NONE',  ( 5.000000000000000000, 6.123233995736766282E-16, 3.000000000000000000 ) ) ;
#7757=FACE_OUTER_BOUND ( 'NONE', #14768, .T. ) ;
#7779=EDGE_CURVE ( 'NONE', #13879, #11517, #6586, .T. ) ;
#7791=ORIENTED_EDGE ( 'NONE', *, *, #17124, .T. ) ;
#7793=ORIENTED_EDGE ( 'NONE', *, *, #18312, .T. ) ;
#7794=PLANE ( 'NONE',  #11745 ) ;
#7804=DIRECTION ( 'NONE',  ( 0.000000000000000000, 0.000000000000000000, -1.000000000000000000 ) ) ;
#7806=EDGE_CURVE ( 'NONE', #16885, #570, #3423, .T. ) ;
#7809=CIRCLE ( 'NONE', #18459, 5.000000000000004441 ) ;
#7849=VECTOR ( 'NONE', #10561, 1000.000000000000000 ) ;
#7868=LINE ( 'NONE', #13580, #6902 ) ;
#7880=ORIENTED_EDGE ( 'NONE', *, *, #16283, .T. ) ;
#7886=CARTESIAN_POINT ( 'NONE',  ( 12.00000000000000711, -19.99999999999999645, 3.000000000000000000 ) ) ;
#7902=CARTESIAN_POINT ( 'NONE',  ( 12.00000000000000711, -14.99999999999999645, 3.000000000000000000 ) ) ;
#7917=EDGE_LOOP ( 'NONE', ( #3096, #16506, #17347, #3298 ) ) ;
#7941=LINE ( 'NONE', #12316, #6710 ) ;
#7952=COLOUR_RGB ( '', 0.66274510, 0.83137255, 0.94901961) ;
#7958=CARTESIAN_POINT ( 'NONE',  ( 6.000000000000001776, 17.00000000000000000, 3.000000000000000000 ) ) ;
#7981=ORIENTED_EDGE ( 'NONE', *, *, #15527, .T. ) ;
#7985=ORIENTED_EDGE ( 'NONE', *, *, #6091, .T. ) ;
#7988=ADVANCED_FACE ( 'NONE', ( #4460, #7242, #3101, #17260 ), #7432, .F. ) ;
#8012=DIRECTION ( 'NONE',  ( 1.000000000000000000, 0.000000000000000000, 0.000000000000000000 ) ) ;
#8036=CARTESIAN_POINT ( 'NONE',  ( -27.32408120756002035, 15.00000000000000000, 0.000000000000000000 ) ) ;
#8061=LINE ( 'NONE', #6529, #6156 ) ;
#8098=AXIS2_PLACEMENT_3D ( 'NONE', #1503, #10096, #11268 ) ;
#8118=CARTESIAN_POINT ( 'NONE',  ( -6.000000000000000888, 17.00000000000000000, 3.000000000000000000 ) ) ;
#8128=CARTESIAN_POINT ( 'NONE',  ( 0.000000000000000000, 0.000000000000000000, 3.000000000000000000 ) ) ;
#8131=MECHANICAL_DESIGN_GEOMETRIC_PRESENTATION_REPRESENTATION('',(#3844),#1719);
#8144=LINE ( 'NONE', #869, #1984 ) ;
#8149=VECTOR ( 'NONE', #6698, 1000.000000000000000 ) ;
#8156=VECTOR ( 'NONE', #16585, 1000.000000000000000 ) ;
#8195=CARTESIAN_POINT ( 'NONE',  ( -59.99999999999997158, -25.00000000000000711, 0.000000000000000000 ) ) ;
#8203=ORIENTED_EDGE ( 'NONE', *, *, #14495, .T. ) ;
#8262=CARTESIAN_POINT ( 'NONE',  ( -27.50000000000000711, -12.50000000000000178, 3.000000000000000000 ) ) ;
#8291=ORIENTED_EDGE ( 'NONE', *, *, #10957, .F. ) ;
#8297=LINE ( 'NONE', #12408, #16377 ) ;
#8317=AXIS2_PLACEMENT_3D ( 'NONE', #10456, #7505, #6160 ) ;
#8319=VERTEX_POINT ( 'NONE', #6203 ) ;
#8341=CARTESIAN_POINT ( 'NONE',  ( -4.000000000000000000, 20.00000000000000000, 8.000000000000000000 ) ) ;
#8350=VECTOR ( 'NONE', #9292, 1000.000000000000000 ) ;
#8358=VERTEX_POINT ( 'NONE', #7656 ) ;
#8369=FILL_AREA_STYLE_COLOUR ( '', #1396 ) ;
#8383=CARTESIAN_POINT ( 'NONE',  ( 12.00000000000000711, -15.99999999999999645, 8.000000000000000000 ) ) ;
#8385=ORIENTED_EDGE ( 'NONE', *, *, #17769, .T. ) ;
#8399=CARTESIAN_POINT ( 'NONE',  ( -30.00000000000000355, -12.50000000000000178, 3.000000000000000000 ) ) ;
#8417=PLANE ( 'NONE',  #2245 ) ;
#8456=VECTOR ( 'NONE', #13583, 1000.000000000000000 ) ;
#8461=DIRECTION ( 'NONE',  ( 0.000000000000000000, 1.000000000000000000, 0.000000000000000000 ) ) ;
#8481=CARTESIAN_POINT ( 'NONE',  ( -194.9999999999999716, -30.00000000000003197, 3.000000000000000000 ) ) ;
#8490=EDGE_CURVE ( 'NONE', #9334, #369, #8297, .T. ) ;
#8499=EDGE_CURVE ( 'NONE', #5275, #3136, #1111, .T. ) ;
#8530=VECTOR ( 'NONE', #12709, 1000.000000000000000 ) ;
#8538=LINE ( 'NONE', #12831, #18225 ) ;
#8566=ADVANCED_FACE ( 'NONE', ( #1589 ), #7243, .T. ) ;
#8585=EDGE_CURVE ( 'NONE', #11329, #1566, #17167, .T. ) ;
#8606=VECTOR ( 'NONE', #12033, 1000.000000000000000 ) ;
#8613=CARTESIAN_POINT ( 'NONE',  ( 14.99999999999999289, 15.00000000000000000, 3.000000000000000000 ) ) ;
#8636=EDGE_LOOP ( 'NONE', ( #278, #2824, #15357, #10482 ) ) ;
#8681=ORIENTED_EDGE ( 'NONE', *, *, #648, .F. ) ;
#8694=AXIS2_PLACEMENT_3D ( 'NONE', #18627, #10127, #2665 ) ;
#8700=LINE ( 'NONE', #4505, #964 ) ;
#8713=CARTESIAN_POINT ( 'NONE',  ( -194.9999999999999716, -45.00000000000003553, 3.000000000000000000 ) ) ;
#8740=DIRECTION ( 'NONE',  ( 1.000000000000000000, -0.000000000000000000, -0.000000000000000000 ) ) ;
#8758=EDGE_LOOP ( 'NONE', ( #9407, #14108, #6423, #13729 ) ) ;
#8772=DIRECTION ( 'NONE',  ( -1.000000000000000000, 0.000000000000000000, 0.000000000000000000 ) ) ;
#8776=DIRECTION ( 'NONE',  ( 1.000000000000000000, 1.577021341797097560E-16, -0.000000000000000000 ) ) ;
#8799=FACE_OUTER_BOUND ( 'NONE', #2438, .T. ) ;
#8802=DIRECTION ( 'NONE',  ( 1.000000000000000000, 0.000000000000000000, 0.000000000000000000 ) ) ;
#8809=EDGE_CURVE ( 'NONE', #5121, #6854, #5663, .T. ) ;
#8814=EDGE_CURVE ( 'NONE', #4000, #6301, #2169, .T. ) ;
#8851=ORIENTED_EDGE ( 'NONE', *, *, #12485, .F. ) ;
#8859=CYLINDRICAL_SURFACE ( 'NONE', #13768, 1.000000000000000000 ) ;
#8885=EDGE_CURVE ( 'NONE', #4825, #5275, #12692, .T. ) ;
#8889=ORIENTED_EDGE ( 'NONE', *, *, #10739, .T. ) ;
#8909=DIRECTION ( 'NONE',  ( 2.891205793294679312E-16, 1.000000000000000000, 0.000000000000000000 ) ) ;
#8915=ORIENTED_EDGE ( 'NONE', *, *, #1710, .F. ) ;
#8918=DIRECTION ( 'NONE',  ( -1.000000000000000000, 0.000000000000000000, 0.000000000000000000 ) ) ;
#8919=CIRCLE ( 'NONE', #5853, 1.000000000000000000 ) ;
#8928=DIRECTION ( 'NONE',  ( 0.000000000000000000, 0.000000000000000000, -1.000000000000000000 ) ) ;
#8940=ORIENTED_EDGE ( 'NONE', *, *, #12536, .F. ) ;
#8944=DIRECTION ( 'NONE',  ( 0.000000000000000000, 0.000000000000000000, -1.000000000000000000 ) ) ;
#8952=CARTESIAN_POINT ( 'NONE',  ( 19.99999999999999645, 15.00000000000000000, 3.000000000000000000 ) ) ;
#8970=CARTESIAN_POINT ( 'NONE',  ( -30.00000000000000355, -12.50000000000000178, 0.000000000000000000 ) ) ;
#8973=ORIENTED_EDGE ( 'NONE', *, *, #1241, .F. ) ;
#9012=CARTESIAN_POINT ( 'NONE',  ( 14.99999999999999289, 15.00000000000000000, 0.000000000000000000 ) ) ;
#9018=ORIENTED_EDGE ( 'NONE', *, *, #5973, .T. ) ;
#9042=VERTEX_POINT ( 'NONE', #15614 ) ;
#9065=AXIS2_PLACEMENT_3D ( 'NONE', #16656, #3461, #10833 ) ;
#9108=DIRECTION ( 'NONE',  ( 0.000000000000000000, 0.000000000000000000, -1.000000000000000000 ) ) ;
#9113=SHAPE_REPRESENTATION ( 'Handle Arm 1', ( #2030 ), #1089 ) ;
#9118=ORIENTED_EDGE ( 'NONE', *, *, #15368, .F. ) ;
#9122=DIRECTION ( 'NONE',  ( -0.000000000000000000, -0.000000000000000000, -1.000000000000000000 ) ) ;
#9135=EDGE_CURVE ( 'NONE', #17750, #16605, #14658, .T. ) ;
#9143=VECTOR ( 'NONE', #753, 1000.000000000000000 ) ;
#9180=ORIENTED_EDGE ( 'NONE', *, *, #12708, .T. ) ;
#9189=VERTEX_POINT ( 'NONE', #15324 ) ;
#9198=LINE ( 'NONE', #317, #17338 ) ;
#9202=CARTESIAN_POINT ( 'NONE',  ( -4.000000000000000888, 17.00000000000000000, 7.000000000000000000 ) ) ;
#9241=EDGE_CURVE ( 'NONE', #9042, #14205, #17245, .T. ) ;
#9255=LINE ( 'NONE', #4677, #6864 ) ;
#9259=ORIENTED_EDGE ( 'NONE', *, *, #11552, .T. ) ;
#9268=EDGE_CURVE ( 'NONE', #4825, #14717, #9411, .T. ) ;
#9280=DIRECTION ( 'NONE',  ( 0.000000000000000000, 0.000000000000000000, -1.000000000000000000 ) ) ;
#9282=ORIENTED_EDGE ( 'NONE', *, *, #18077, .F. ) ;
#9292=DIRECTION ( 'NONE',  ( -1.000000000000000000, -1.734723475976807094E-16, 0.000000000000000000 ) ) ;
#9294=DIRECTION ( 'NONE',  ( -1.000000000000000000, 0.000000000000000000, 0.000000000000000000 ) ) ;
#9296=VERTEX_POINT ( 'NONE', #7902 ) ;
#9300=FACE_OUTER_BOUND ( 'NONE', #7159, .T. ) ;
#9313=CARTESIAN_POINT ( 'NONE',  ( 7.000000000000000000, 8.572527594031473190E-16, 3.000000000000000000 ) ) ;
#9325=AXIS2_PLACEMENT_3D ( 'NONE', #18771, #8461, #6944 ) ;
#9334=VERTEX_POINT ( 'NONE', #12916 ) ;
#9353=VECTOR ( 'NONE', #7289, 1000.000000000000000 ) ;
#9372=AXIS2_PLACEMENT_3D ( 'NONE', #16158, #2850, #17491 ) ;
#9374=ORIENTED_EDGE ( 'NONE', *, *, #5158, .F. ) ;
#9398=ORIENTED_EDGE ( 'NONE', *, *, #16532, .T. ) ;
#9400=CARTESIAN_POINT ( 'NONE',  ( 4.000000000000006217, 1.156482317317873500E-15, 7.000000000000000000 ) ) ;
#9407=ORIENTED_EDGE ( 'NONE', *, *, #5004, .T. ) ;
#9411=LINE ( 'NONE', #9586, #10548 ) ;
#9441=CARTESIAN_POINT ( 'NONE',  ( 14.99999999999999289, 15.00000000000000000, 3.000000000000000000 ) ) ;
#9463=MECHANICAL_DESIGN_GEOMETRIC_PRESENTATION_REPRESENTATION('',(#17705),#1202);
#9465=ADVANCED_FACE ( 'NONE', ( #6046 ), #313, .F. ) ;
#9494=CARTESIAN_POINT ( 'NONE',  ( -59.99999999999997158, -25.00000000000000711, 3.000000000000000000 ) ) ;
#9498=DIRECTION ( 'NONE',  ( 0.000000000000000000, 0.000000000000000000, -1.000000000000000000 ) ) ;
#9501=PRODUCT_CONTEXT ( 'NONE', #12898, 'mechanical' ) ;
#9502=EDGE_CURVE ( 'NONE', #16237, #14846, #17866, .T. ) ;
#9569=FACE_BOUND ( 'NONE', #1226, .T. ) ;
#9586=CARTESIAN_POINT ( 'NONE',  ( 15.00000000000000711, -14.99999999999999645, 8.000000000000000000 ) ) ;
#9593=DIRECTION ( 'NONE',  ( 0.000000000000000000, 1.000000000000000000, 0.000000000000000000 ) ) ;
#9598=EDGE_CURVE ( 'NONE', #15937, #11936, #2036, .T. ) ;
#9601=AXIS2_PLACEMENT_3D ( 'NONE', #5682, #15629, #7241 ) ;
#9608=AXIS2_PLACEMENT_3D ( 'NONE', #7388, #4519, #1743 ) ;
#9618=ORIENTED_EDGE ( 'NONE', *, *, #12485, .T. ) ;
#9687=SHAPE_DEFINITION_REPRESENTATION ( #16065, #9113 ) ;
#9706=EDGE_CURVE ( 'NONE', #13879, #16287, #16353, .T. ) ;
#9728=DIRECTION ( 'NONE',  ( -1.000000000000000000, 0.000000000000000000, 0.000000000000000000 ) ) ;
#9739=AXIS2_PLACEMENT_3D ( 'NONE', #4409, #17313, #4131 ) ;
#9756=LINE ( 'NONE', #14258, #9808 ) ;
#9758=ADVANCED_FACE ( 'NONE', ( #2390 ), #6991, .F. ) ;
#9773=CARTESIAN_POINT ( 'NONE',  ( -5.000000000000000000, 20.00000000000000000, 8.000000000000000000 ) ) ;
#9775=DIRECTION ( 'NONE',  ( 1.000000000000000000, 1.577021341797097560E-16, -0.000000000000000000 ) ) ;
#9783=CARTESIAN_POINT ( 'NONE',  ( 6.000000000000000000, 20.00000000000000000, 4.000000000000000000 ) ) ;
#9794=ORIENTED_EDGE ( 'NONE', *, *, #5211, .F. ) ;
#9808=VECTOR ( 'NONE', #17598, 1000.000000000000000 ) ;
#9828=ORIENTED_EDGE ( 'NONE', *, *, #4942, .F. ) ;
#9852=DIRECTION ( 'NONE',  ( -1.000000000000000000, 0.000000000000000000, 0.000000000000000000 ) ) ;
#9870=VECTOR ( 'NONE', #16904, 1000.000000000000000 ) ;
#9892=ORIENTED_EDGE ( 'NONE', *, *, #15265, .T. ) ;
#9894=ORIENTED_EDGE ( 'NONE', *, *, #11552, .F. ) ;
#9903=ORIENTED_EDGE ( 'NONE', *, *, #5699, .T. ) ;
#9905=AXIS2_PLACEMENT_3D ( 'NONE', #8970, #13078, #13369 ) ;
#9911=FACE_OUTER_BOUND ( 'NONE', #10358, .T. ) ;
#9931=AXIS2_PLACEMENT_3D ( 'NONE', #10173, #44, #8928 ) ;
#9933=AXIS2_PLACEMENT_3D ( 'NONE', #5058, #18251, #10997 ) ;
#9948=DIRECTION ( 'NONE',  ( -0.000000000000000000, -0.000000000000000000, 1.000000000000000000 ) ) ;
#9951=CARTESIAN_POINT ( 'NONE',  ( -32.49999999999999289, -12.50000000000000178, 0.000000000000000000 ) ) ;
#9958=AXIS2_PLACEMENT_3D ( 'NONE', #16104, #14854, #6164 ) ;
#10000=ADVANCED_FACE ( 'NONE', ( #11427 ), #18397, .T. ) ;
#10050=CARTESIAN_POINT ( 'NONE',  ( -199.9999999999999716, -40.00000000000003553, 3.000000000000000000 ) ) ;
#10055=LINE ( 'NONE', #8262, #13016 ) ;
#10063=PLANE ( 'NONE',  #18530 ) ;
#10071=CARTESIAN_POINT ( 'NONE',  ( 12.00000000000000711, -15.99999999999999645, 7.000000000000000000 ) ) ;
#10081=SURFACE_STYLE_FILL_AREA ( #17065 ) ;
#10087=ORIENTED_EDGE ( 'NONE', *, *, #5973, .F. ) ;
#10090=ORIENTED_EDGE ( 'NONE', *, *, #5975, .T. ) ;
#10096=DIRECTION ( 'NONE',  ( 1.000000000000000000, 0.000000000000000000, 0.000000000000000000 ) ) ;
#10102=DIRECTION ( 'NONE',  ( -0.000000000000000000, -0.000000000000000000, -1.000000000000000000 ) ) ;
#10115=EDGE_CURVE ( 'NONE', #9334, #4587, #4440, .T. ) ;
#10127=DIRECTION ( 'NONE',  ( 1.000000000000000000, 0.000000000000000000, 0.000000000000000000 ) ) ;
#10135=LINE ( 'NONE', #7184, #6771 ) ;
#10173=CARTESIAN_POINT ( 'NONE',  ( 4.000000000000000000, 20.00000000000000000, 7.000000000000000000 ) ) ;
#10191=DIRECTION ( 'NONE',  ( 1.000000000000000000, 0.000000000000000000, 0.000000000000000000 ) ) ;
#10200=CARTESIAN_POINT ( 'NONE',  ( 20.00000000000000711, -45.00000000000000000, 3.000000000000000000 ) ) ;
#10254=DIRECTION ( 'NONE',  ( -0.000000000000000000, -0.000000000000000000, 1.000000000000000000 ) ) ;
#10280=CYLINDRICAL_SURFACE ( 'NONE', #17293, 5.000000000000004441 ) ;
#10288=DIRECTION ( 'NONE',  ( -1.000000000000000000, 0.000000000000000000, -0.000000000000000000 ) ) ;
#10328=DIRECTION ( 'NONE',  ( -0.000000000000000000, -0.000000000000000000, 1.000000000000000000 ) ) ;
#10343=DIRECTION ( 'NONE',  ( -1.000000000000000000, 0.000000000000000000, 0.000000000000000000 ) ) ;
#10349=CARTESIAN_POINT ( 'NONE',  ( 0.000000000000000000, 0.000000000000000000, 8.000000000000000000 ) ) ;
#10358=EDGE_LOOP ( 'NONE', ( #93, #9180, #11675, #16418 ) ) ;
#10361=AXIS2_PLACEMENT_3D ( 'NONE', #1432, #7272, #13084 ) ;
#10397=ORIENTED_EDGE ( 'NONE', *, *, #5158, .T. ) ;
#10445=DIRECTION ( 'NONE',  ( -1.000000000000000000, 0.000000000000000000, 0.000000000000000000 ) ) ;
#10454=EDGE_CURVE ( 'NONE', #14846, #7133, #11089, .T. ) ;
#10456=CARTESIAN_POINT ( 'NONE',  ( 0.000000000000000000, 0.000000000000000000, 3.000000000000000000 ) ) ;
#10477=ADVANCED_FACE ( 'NONE', ( #18252 ), #10711, .T. ) ;
#10482=ORIENTED_EDGE ( 'NONE', *, *, #15527, .F. ) ;
#10548=VECTOR ( 'NONE', #10753, 1000.000000000000000 ) ;
#10559=( NAMED_UNIT ( * ) SI_UNIT ( $, .STERADIAN. ) SOLID_ANGLE_UNIT ( ) );
#10561=DIRECTION ( 'NONE',  ( 2.891205793294679312E-16, 1.000000000000000000, -0.000000000000000000 ) ) ;
#10588=CARTESIAN_POINT ( 'NONE',  ( 12.00000000000000711, -19.99999999999999645, 7.000000000000000000 ) ) ;
#10607=CARTESIAN_POINT ( 'NONE',  ( 5.999999999999998224, 20.00000000000000000, 3.000000000000000000 ) ) ;
#10648=VERTEX_POINT ( 'NONE', #1310 ) ;
#10691=CARTESIAN_POINT ( 'NONE',  ( 15.00000000000000711, -45.00000000000000000, 3.000000000000000000 ) ) ;
#10710=DIRECTION ( 'NONE',  ( 0.000000000000000000, 1.000000000000000000, 0.000000000000000000 ) ) ;
#10711=CYLINDRICAL_SURFACE ( 'NONE', #2806, 7.000000000000000000 ) ;
#10735=FACE_OUTER_BOUND ( 'NONE', #13191, .T. ) ;
#10739=EDGE_CURVE ( 'NONE', #4587, #5121, #4471, .T. ) ;
#10745=ORIENTED_EDGE ( 'NONE', *, *, #8499, .T. ) ;
#10753=DIRECTION ( 'NONE',  ( -0.000000000000000000, -0.000000000000000000, -1.000000000000000000 ) ) ;
#10755=PRODUCT ( 'Handle Arm 1', 'Handle Arm 1', '', ( #9501 ) ) ;
#10783=CARTESIAN_POINT ( 'NONE',  ( 0.000000000000000000, 0.000000000000000000, 8.000000000000000000 ) ) ;
#10808=ORIENTED_EDGE ( 'NONE', *, *, #8490, .T. ) ;
#10819=CARTESIAN_POINT ( 'NONE',  ( -30.00000000000000711, 20.00000000000000000, 0.000000000000000000 ) ) ;
#10831=EDGE_CURVE ( 'NONE', #14846, #16237, #95, .T. ) ;
#10833=DIRECTION ( 'NONE',  ( -1.000000000000000000, -1.577021341797097560E-16, 0.000000000000000000 ) ) ;
#10840=AXIS2_PLACEMENT_3D ( 'NONE', #15925, #2725, #10191 ) ;
#10841=ORIENTED_EDGE ( 'NONE', *, *, #6601, .F. ) ;
#10845=ADVANCED_BREP_SHAPE_REPRESENTATION ( '', ( #3589, #2030 ), #1089 ) ;
#10860=AXIS2_PLACEMENT_3D ( 'NONE', #12614, #6262, #14059 ) ;
#10888=VECTOR ( 'NONE', #2812, 1000.000000000000000 ) ;
#10899=DIRECTION ( 'NONE',  ( 0.000000000000000000, 0.000000000000000000, -1.000000000000000000 ) ) ;
#10949=CARTESIAN_POINT ( 'NONE',  ( 12.00000000000000711, -19.99999999999999645, 7.000000000000000000 ) ) ;
#10957=EDGE_CURVE ( 'NONE', #11716, #10648, #3783, .T. ) ;
#10977=DIRECTION ( 'NONE',  ( -2.891205793294679312E-16, -1.000000000000000000, 0.000000000000000000 ) ) ;
#10978=EDGE_LOOP ( 'NONE', ( #4651, #17317, #9118, #14284 ) ) ;
#10981=ORIENTED_EDGE ( 'NONE', *, *, #2827, .F. ) ;
#10997=DIRECTION ( 'NONE',  ( -1.000000000000000000, 0.000000000000000000, 0.000000000000000000 ) ) ;
#11026=CARTESIAN_POINT ( 'NONE',  ( -27.50000000000000711, -12.50000000000000178, 0.000000000000000000 ) ) ;
#11028=ORIENTED_EDGE ( 'NONE', *, *, #8809, .F. ) ;
#11031=DIRECTION ( 'NONE',  ( 1.000000000000000000, 1.734723475976806848E-16, 0.000000000000000000 ) ) ;
#11075=LINE ( 'NONE', #5320, #17859 ) ;
#11089=LINE ( 'NONE', #5059, #9870 ) ;
#11121=ORIENTED_EDGE ( 'NONE', *, *, #13472, .F. ) ;
#11140=VECTOR ( 'NONE', #12139, 1000.000000000000000 ) ;
#11145=DIRECTION ( 'NONE',  ( 0.000000000000000000, -1.000000000000000000, 0.000000000000000000 ) ) ;
#11248=DIRECTION ( 'NONE',  ( 0.000000000000000000, 0.000000000000000000, 1.000000000000000000 ) ) ;
#11268=DIRECTION ( 'NONE',  ( 0.000000000000000000, 0.000000000000000000, -1.000000000000000000 ) ) ;
#11294=DIRECTION ( 'NONE',  ( 1.000000000000000000, 0.000000000000000000, -0.000000000000000000 ) ) ;
#11316=ORIENTED_EDGE ( 'NONE', *, *, #9241, .F. ) ;
#11323=DIRECTION ( 'NONE',  ( 0.000000000000000000, 0.000000000000000000, 1.000000000000000000 ) ) ;
#11329=VERTEX_POINT ( 'NONE', #15602 ) ;
#11381=DIRECTION ( 'NONE',  ( 1.000000000000000000, 0.000000000000000000, 0.000000000000000000 ) ) ;
#11384=DIRECTION ( 'NONE',  ( 0.000000000000000000, 0.000000000000000000, 1.000000000000000000 ) ) ;
#11427=FACE_OUTER_BOUND ( 'NONE', #3813, .T. ) ;
#11435=ORIENTED_EDGE ( 'NONE', *, *, #2680, .F. ) ;
#11440=DIRECTION ( 'NONE',  ( 0.000000000000000000, 0.000000000000000000, 1.000000000000000000 ) ) ;
#11514=ORIENTED_EDGE ( 'NONE', *, *, #3045, .F. ) ;
#11517=VERTEX_POINT ( 'NONE', #7594 ) ;
#11549=PLANE ( 'NONE',  #952 ) ;
#11552=EDGE_CURVE ( 'NONE', #570, #18779, #4903, .T. ) ;
#11557=ORIENTED_EDGE ( 'NONE', *, *, #18545, .F. ) ;
#11634=PRODUCT_DEFINITION ( 'UNKNOWN', '', #12039, #1 ) ;
#11675=ORIENTED_EDGE ( 'NONE', *, *, #15265, .F. ) ;
#11691=ADVANCED_FACE ( 'NONE', ( #5175 ), #8417, .F. ) ;
#11715=DIRECTION ( 'NONE',  ( -1.000000000000000000, 0.000000000000000000, 0.000000000000000000 ) ) ;
#11716=VERTEX_POINT ( 'NONE', #5265 ) ;
#11745=AXIS2_PLACEMENT_3D ( 'NONE', #9494, #12184, #11031 ) ;
#11746=ORIENTED_EDGE ( 'NONE', *, *, #18071, .T. ) ;
#11768=CARTESIAN_POINT ( 'NONE',  ( 0.000000000000000000, 0.000000000000000000, 0.000000000000000000 ) ) ;
#11788=CIRCLE ( 'NONE', #2033, 5.000000000000000888 ) ;
#11794=ORIENTED_EDGE ( 'NONE', *, *, #8814, .F. ) ;
#11809=CARTESIAN_POINT ( 'NONE',  ( 6.000000000000000888, 17.00000000000000000, 3.000000000000000000 ) ) ;
#11871=FACE_OUTER_BOUND ( 'NONE', #2878, .T. ) ;
#11882=FACE_OUTER_BOUND ( 'NONE', #18623, .T. ) ;
#11888=CARTESIAN_POINT ( 'NONE',  ( 15.00000000000000711, -14.99999999999999645, 7.000000000000000000 ) ) ;
#11911=ORIENTED_EDGE ( 'NONE', *, *, #9268, .F. ) ;
#11936=VERTEX_POINT ( 'NONE', #17786 ) ;
#11961=DIRECTION ( 'NONE',  ( -1.000000000000000000, -0.000000000000000000, -0.000000000000000000 ) ) ;
#11983=EDGE_LOOP ( 'NONE', ( #17492, #1011, #16615, #423, #15354, #6442 ) ) ;
#11984=ORIENTED_EDGE ( 'NONE', *, *, #7806, .T. ) ;
#12033=DIRECTION ( 'NONE',  ( 1.000000000000000000, 0.000000000000000000, 0.000000000000000000 ) ) ;
#12039=PRODUCT_DEFINITION_FORMATION_WITH_SPECIFIED_SOURCE ( 'ANY', '', #10755, .NOT_KNOWN. ) ;
#12051=ORIENTED_EDGE ( 'NONE', *, *, #6850, .T. ) ;
#12065=AXIS2_PLACEMENT_3D ( 'NONE', #17200, #4111, #12611 ) ;
#12072=EDGE_CURVE ( 'NONE', #6854, #5564, #5868, .T. ) ;
#12078=CARTESIAN_POINT ( 'NONE',  ( -5.000000000000000000, 0.000000000000000000, 3.000000000000000000 ) ) ;
#12080=ORIENTED_EDGE ( 'NONE', *, *, #14495, .F. ) ;
#12087=VERTEX_POINT ( 'NONE', #3287 ) ;
#12139=DIRECTION ( 'NONE',  ( -0.000000000000000000, -0.000000000000000000, -1.000000000000000000 ) ) ;
#12184=DIRECTION ( 'NONE',  ( 1.734723475976806848E-16, -1.000000000000000000, 0.000000000000000000 ) ) ;
#12205=ORIENTED_EDGE ( 'NONE', *, *, #17769, .F. ) ;
#12252=VERTEX_POINT ( 'NONE', #18384 ) ;
#12253=CARTESIAN_POINT ( 'NONE',  ( 12.00000000000000711, -14.99999999999999645, 7.000000000000000000 ) ) ;
#12267=ORIENTED_EDGE ( 'NONE', *, *, #560, .F. ) ;
#12271=CARTESIAN_POINT ( 'NONE',  ( 15.00000000000000711, -14.99999999999999645, 8.000000000000000000 ) ) ;
#12316=CARTESIAN_POINT ( 'NONE',  ( 14.99999999999999289, 20.00000000000000000, 3.000000000000000000 ) ) ;
#12363=SURFACE_STYLE_FILL_AREA ( #626 ) ;
#12375=VECTOR ( 'NONE', #12522, 1000.000000000000000 ) ;
#12395=LINE ( 'NONE', #18230, #6010 ) ;
#12408=CARTESIAN_POINT ( 'NONE',  ( -5.000000000000000000, 20.00000000000000000, 8.000000000000000000 ) ) ;
#12426=CARTESIAN_POINT ( 'NONE',  ( 5.000000000000000888, 17.00000000000000000, 7.000000000000000000 ) ) ;
#12430=CLOSED_SHELL ( 'NONE', ( #10477, #18464, #2802, #7988, #12612, #1660, #7326, #4074, #5239, #13336, #18009, #5511, #7201, #5779, #2204, #18531, #13703, #12512, #1224, #7284, #9758, #11691, #2569, #15362, #18289, #3727, #2112, #13035, #2130, #3097, #9465, #16503, #8566, #10000, #15427 ) ) ;
#12454=ORIENTED_EDGE ( 'NONE', *, *, #7200, .F. ) ;
#12460=CARTESIAN_POINT ( 'NONE',  ( -199.9999999999999716, -40.00000000000003553, 3.000000000000000000 ) ) ;
#12485=EDGE_CURVE ( 'NONE', #6301, #14205, #8061, .T. ) ;
#12505=DIRECTION ( 'NONE',  ( -0.000000000000000000, -0.000000000000000000, -1.000000000000000000 ) ) ;
#12509=CARTESIAN_POINT ( 'NONE',  ( -194.9999999999999716, -40.00000000000003553, 3.000000000000000000 ) ) ;
#12512=ADVANCED_FACE ( 'NONE', ( #10735 ), #6433, .T. ) ;
#12522=DIRECTION ( 'NONE',  ( -0.000000000000000000, -0.000000000000000000, -1.000000000000000000 ) ) ;
#12536=EDGE_CURVE ( 'NONE', #2858, #18187, #16221, .T. ) ;
#12590=CARTESIAN_POINT ( 'NONE',  ( 6.000000000000000000, 20.00000000000000000, 4.000000000000000000 ) ) ;
#12611=DIRECTION ( 'NONE',  ( 1.000000000000000000, 0.000000000000000000, 0.000000000000000000 ) ) ;
#12612=ADVANCED_FACE ( 'NONE', ( #17030, #9569, #18362 ), #17205, .T. ) ;
#12614=CARTESIAN_POINT ( 'NONE',  ( -30.00000000000000711, 20.00000000000000000, 3.000000000000000000 ) ) ;
#12634=FACE_OUTER_BOUND ( 'NONE', #8636, .T. ) ;
#12647=DIRECTION ( 'NONE',  ( -1.601283208593975514E-16, 1.000000000000000000, -0.000000000000000000 ) ) ;
#12663=CIRCLE ( 'NONE', #474, 5.000000000000000000 ) ;
#12665=( NAMED_UNIT ( * ) PLANE_ANGLE_UNIT ( ) SI_UNIT ( $, .RADIAN. ) );
#12668=EDGE_CURVE ( 'NONE', #12087, #11329, #15303, .T. ) ;
#12692=CIRCLE ( 'NONE', #7222, 1.000000000000000000 ) ;
#12696=DIRECTION ( 'NONE',  ( 0.000000000000000000, 0.000000000000000000, 1.000000000000000000 ) ) ;
#12708=EDGE_CURVE ( 'NONE', #14346, #12958, #10135, .T. ) ;
#12709=DIRECTION ( 'NONE',  ( -2.891205793294679312E-16, -1.000000000000000000, 0.000000000000000000 ) ) ;
#12749=EDGE_CURVE ( 'NONE', #6964, #16555, #198, .T. ) ;
#12759=( LENGTH_UNIT ( ) NAMED_UNIT ( * ) SI_UNIT ( .MILLI., .METRE. ) );
#12786=CARTESIAN_POINT ( 'NONE',  ( -194.9999999999999716, -40.00000000000003553, 3.000000000000000000 ) ) ;
#12795=EDGE_CURVE ( 'NONE', #8319, #5753, #8700, .T. ) ;
#12831=CARTESIAN_POINT ( 'NONE',  ( 19.99999999999999645, 20.00000000000000000, 3.000000000000000000 ) ) ;
#12865=DIRECTION ( 'NONE',  ( -1.000000000000000000, 0.000000000000000000, 0.000000000000000000 ) ) ;
#12880=EDGE_LOOP ( 'NONE', ( #1429, #1828, #16159, #14850 ) ) ;
#12897=CARTESIAN_POINT ( 'NONE',  ( 15.00000000000000711, -45.00000000000000000, 0.000000000000000000 ) ) ;
#12898=APPLICATION_CONTEXT ( 'automotive_design' ) ;
#12903=EDGE_CURVE ( 'NONE', #2858, #14346, #4279, .T. ) ;
#12916=CARTESIAN_POINT ( 'NONE',  ( 4.000000000000000888, 20.00000000000000000, 8.000000000000000000 ) ) ;
#12955=PLANE ( 'NONE',  #6258 ) ;
#12956=CIRCLE ( 'NONE', #6268, 1.000000000000000000 ) ;
#12958=VERTEX_POINT ( 'NONE', #8952 ) ;
#12968=CARTESIAN_POINT ( 'NONE',  ( 15.00000000000000711, -19.99999999999999645, 8.000000000000000000 ) ) ;
#12977=EDGE_CURVE ( 'NONE', #5607, #1182, #5992, .T. ) ;
#12999=AXIS2_PLACEMENT_3D ( 'NONE', #9783, #11145, #14006 ) ;
#13016=VECTOR ( 'NONE', #4134, 1000.000000000000000 ) ;
#13025=CARTESIAN_POINT ( 'NONE',  ( 15.00000000000000711, -18.99999999999999645, 7.000000000000000000 ) ) ;
#13035=ADVANCED_FACE ( 'NONE', ( #7250 ), #8859, .T. ) ;
#13043=DIRECTION ( 'NONE',  ( -1.000000000000000000, -0.000000000000000000, -0.000000000000000000 ) ) ;
#13049=ORIENTED_EDGE ( 'NONE', *, *, #5699, .F. ) ;
#13054=LINE ( 'NONE', #5588, #16930 ) ;
#13056=DIRECTION ( 'NONE',  ( -1.000000000000000000, 2.891205793294679805E-16, 0.000000000000000000 ) ) ;
#13061=DIRECTION ( 'NONE',  ( 0.000000000000000000, 0.000000000000000000, 1.000000000000000000 ) ) ;
#13078=DIRECTION ( 'NONE',  ( 0.000000000000000000, 0.000000000000000000, 1.000000000000000000 ) ) ;
#13084=DIRECTION ( 'NONE',  ( -0.000000000000000000, 0.000000000000000000, -1.000000000000000000 ) ) ;
#13103=DIRECTION ( 'NONE',  ( 0.000000000000000000, 0.000000000000000000, 1.000000000000000000 ) ) ;
#13130=EDGE_LOOP ( 'NONE', ( #9282, #14, #1608, #7375 ) ) ;
#13135=PLANE ( 'NONE',  #9958 ) ;
#13147=ORIENTED_EDGE ( 'NONE', *, *, #1710, .T. ) ;
#13153=FACE_OUTER_BOUND ( 'NONE', #7917, .T. ) ;
#13177=ORIENTED_EDGE ( 'NONE', *, *, #14767, .F. ) ;
#13184=ORIENTED_EDGE ( 'NONE', *, *, #4942, .T. ) ;
#13191=EDGE_LOOP ( 'NONE', ( #1759, #8973, #8940, #1724 ) ) ;
#13193=UNCERTAINTY_MEASURE_WITH_UNIT (LENGTH_MEASURE( 1.000000000000000082E-05 ), #14378, 'distance_accuracy_value', 'NONE');
#13312=CARTESIAN_POINT ( 'NONE',  ( -5.000000000000000000, 0.000000000000000000, 8.000000000000000000 ) ) ;
#13336=ADVANCED_FACE ( 'NONE', ( #9911 ), #11549, .F. ) ;
#13354=CARTESIAN_POINT ( 'NONE',  ( 0.000000000000000000, -18.99999999999999645, 7.000000000000000000 ) ) ;
#13359=LINE ( 'NONE', #7646, #2635 ) ;
#13361=VERTEX_POINT ( 'NONE', #14039 ) ;
#13369=DIRECTION ( 'NONE',  ( 1.000000000000000000, 0.000000000000000000, 0.000000000000000000 ) ) ;
#13403=DIRECTION ( 'NONE',  ( -1.000000000000000000, -0.000000000000000000, -0.000000000000000000 ) ) ;
#13460=CARTESIAN_POINT ( 'NONE',  ( -30.00000000000000711, 20.00000000000000000, 3.000000000000000000 ) ) ;
#13461=DIRECTION ( 'NONE',  ( -0.000000000000000000, -0.000000000000000000, 1.000000000000000000 ) ) ;
#13472=EDGE_CURVE ( 'NONE', #14717, #9296, #16029, .T. ) ;
#13481=EDGE_LOOP ( 'NONE', ( #704, #15408, #9018, #17721 ) ) ;
#13489=EDGE_CURVE ( 'NONE', #14463, #18838, #1600, .T. ) ;
#13508=FACE_OUTER_BOUND ( 'NONE', #14460, .T. ) ;
#13541=VECTOR ( 'NONE', #7422, 1000.000000000000000 ) ;
#13550=EDGE_LOOP ( 'NONE', ( #13049, #16315 ) ) ;
#13580=CARTESIAN_POINT ( 'NONE',  ( 5.000000000000000000, 20.00000000000000000, 4.000000000000000000 ) ) ;
#13583=DIRECTION ( 'NONE',  ( -0.5547001962252284812, -0.8320502943378440541, 0.000000000000000000 ) ) ;
#13594=CARTESIAN_POINT ( 'NONE',  ( 15.00000000000000711, -39.99999999999999289, 3.000000000000000000 ) ) ;
#13606=DIRECTION ( 'NONE',  ( 1.000000000000000000, -0.000000000000000000, -0.000000000000000000 ) ) ;
#13615=LINE ( 'NONE', #10949, #7235 ) ;
#13643=CIRCLE ( 'NONE', #1417, 2.499999999999995115 ) ;
#13658=ORIENTED_EDGE ( 'NONE', *, *, #7688, .F. ) ;
#13659=VECTOR ( 'NONE', #9775, 1000.000000000000000 ) ;
#13662=AXIS2_PLACEMENT_3D ( 'NONE', #9202, #16658, #18003 ) ;
#13667=VERTEX_POINT ( 'NONE', #16704 ) ;
#13679=ORIENTED_EDGE ( 'NONE', *, *, #5746, .F. ) ;
#13698=EDGE_LOOP ( 'NONE', ( #16596, #5637 ) ) ;
#13703=ADVANCED_FACE ( 'NONE', ( #6479 ), #3606, .T. ) ;
#13710=FILL_AREA_STYLE_COLOUR ( '', #7952 ) ;
#13729=ORIENTED_EDGE ( 'NONE', *, *, #9135, .T. ) ;
#13768=AXIS2_PLACEMENT_3D ( 'NONE', #13354, #8772, #13061 ) ;
#13776=APPLICATION_CONTEXT ( 'automotive_design' ) ;
#13787=CARTESIAN_POINT ( 'NONE',  ( -4.000000000000000000, 20.00000000000000000, 7.000000000000000000 ) ) ;
#13798=CARTESIAN_POINT ( 'NONE',  ( 15.00000000000000711, -18.99999999999999645, 8.000000000000000000 ) ) ;
#13808=ORIENTED_EDGE ( 'NONE', *, *, #7200, .T. ) ;
#13877=ORIENTED_EDGE ( 'NONE', *, *, #15551, .F. ) ;
#13878=AXIS2_PLACEMENT_3D ( 'NONE', #8481, #14310, #12865 ) ;
#13879=VERTEX_POINT ( 'NONE', #7324 ) ;
#13884=CIRCLE ( 'NONE', #9905, 2.499999999999995115 ) ;
#13893=EDGE_CURVE ( 'NONE', #6155, #8319, #1387, .T. ) ;
#13940=DIRECTION ( 'NONE',  ( -1.000000000000000000, 0.000000000000000000, 0.000000000000000000 ) ) ;
#13953=ORIENTED_EDGE ( 'NONE', *, *, #9268, .T. ) ;
#13967=CARTESIAN_POINT ( 'NONE',  ( -30.00000000000000355, -12.50000000000000178, 3.000000000000000000 ) ) ;
#14006=DIRECTION ( 'NONE',  ( 0.000000000000000000, 0.000000000000000000, -1.000000000000000000 ) ) ;
#14036=CYLINDRICAL_SURFACE ( 'NONE', #5062, 2.499999999999992006 ) ;
#14039=CARTESIAN_POINT ( 'NONE',  ( 12.00000000000000711, -18.99999999999999645, 8.000000000000000000 ) ) ;
#14042=CARTESIAN_POINT ( 'NONE',  ( -27.32408120756002035, 20.00000000000000000, 3.000000000000000000 ) ) ;
#14059=DIRECTION ( 'NONE',  ( 0.000000000000000000, -0.000000000000000000, -1.000000000000000000 ) ) ;
#14079=DIRECTION ( 'NONE',  ( -1.000000000000000000, 0.000000000000000000, 0.000000000000000000 ) ) ;
#14108=ORIENTED_EDGE ( 'NONE', *, *, #14767, .T. ) ;
#14109=CARTESIAN_POINT ( 'NONE',  ( 15.00000000000000711, -19.99999999999999645, 8.000000000000000000 ) ) ;
#14111=DIRECTION ( 'NONE',  ( -1.000000000000000000, -0.000000000000000000, -0.000000000000000000 ) ) ;
#14123=DIRECTION ( 'NONE',  ( 0.000000000000000000, 1.000000000000000000, 0.000000000000000000 ) ) ;
#14126=CARTESIAN_POINT ( 'NONE',  ( 0.000000000000000000, 0.000000000000000000, 8.000000000000000000 ) ) ;
#14165=CARTESIAN_POINT ( 'NONE',  ( 20.00000000000000711, -39.99999999999999289, 0.000000000000000000 ) ) ;
#14205=VERTEX_POINT ( 'NONE', #222 ) ;
#14228=DIRECTION ( 'NONE',  ( -1.000000000000000000, 0.000000000000000000, 0.000000000000000000 ) ) ;
#14255=EDGE_LOOP ( 'NONE', ( #9828, #2254, #6579, #11794 ) ) ;
#14258=CARTESIAN_POINT ( 'NONE',  ( 5.000000000000000888, 17.00000000000000000, 7.000000000000000000 ) ) ;
#14271=DIRECTION ( 'NONE',  ( -0.000000000000000000, -0.000000000000000000, -1.000000000000000000 ) ) ;
#14284=ORIENTED_EDGE ( 'NONE', *, *, #3436, .F. ) ;
#14289=DIRECTION ( 'NONE',  ( 0.000000000000000000, 0.000000000000000000, 1.000000000000000000 ) ) ;
#14296=PRESENTATION_STYLE_ASSIGNMENT (( #15814 ) ) ;
#14305=ORIENTED_EDGE ( 'NONE', *, *, #9502, .F. ) ;
#14310=DIRECTION ( 'NONE',  ( 0.000000000000000000, 0.000000000000000000, -1.000000000000000000 ) ) ;
#14312=EDGE_CURVE ( 'NONE', #3136, #13361, #9198, .T. ) ;
#14321=ORIENTED_EDGE ( 'NONE', *, *, #10831, .F. ) ;
#14330=CARTESIAN_POINT ( 'NONE',  ( 15.00000000000000711, -14.99999999999999645, 7.000000000000000000 ) ) ;
#14346=VERTEX_POINT ( 'NONE', #16906 ) ;
#14378=( LENGTH_UNIT ( ) NAMED_UNIT ( * ) SI_UNIT ( .MILLI., .METRE. ) );
#14403=CARTESIAN_POINT ( 'NONE',  ( -194.9999999999999716, -45.00000000000003553, 3.000000000000000000 ) ) ;
#14405=VERTEX_POINT ( 'NONE', #17006 ) ;
#14460=EDGE_LOOP ( 'NONE', ( #10981, #5412, #2230, #3848 ) ) ;
#14463=VERTEX_POINT ( 'NONE', #14403 ) ;
#14471=( NAMED_UNIT ( * ) SI_UNIT ( $, .STERADIAN. ) SOLID_ANGLE_UNIT ( ) );
#14474=VECTOR ( 'NONE', #11961, 1000.000000000000000 ) ;
#14480=ORIENTED_EDGE ( 'NONE', *, *, #5004, .F. ) ;
#14495=EDGE_CURVE ( 'NONE', #2604, #5275, #2732, .T. ) ;
#14508=ORIENTED_EDGE ( 'NONE', *, *, #10454, .T. ) ;
#14510=ORIENTED_EDGE ( 'NONE', *, *, #16024, .T. ) ;
#14538=LINE ( 'NONE', #8713, #3576 ) ;
#14585=DIRECTION ( 'NONE',  ( -1.000000000000000000, 1.387778780781445478E-15, 0.000000000000000000 ) ) ;
#14619=CARTESIAN_POINT ( 'NONE',  ( -6.000000000000000000, 20.00000000000000000, 3.000000000000000000 ) ) ;
#14626=EDGE_CURVE ( 'NONE', #1746, #9296, #13359, .T. ) ;
#14646=ORIENTED_EDGE ( 'NONE', *, *, #2129, .T. ) ;
#14647=CARTESIAN_POINT ( 'NONE',  ( 14.99999999999999289, 20.00000000000000000, 0.000000000000000000 ) ) ;
#14658=LINE ( 'NONE', #17926, #7849 ) ;
#14669=DIRECTION ( 'NONE',  ( -0.000000000000000000, -0.000000000000000000, 1.000000000000000000 ) ) ;
#14673=VERTEX_POINT ( 'NONE', #3608 ) ;
#14703=ORIENTED_EDGE ( 'NONE', *, *, #8490, .F. ) ;
#14717=VERTEX_POINT ( 'NONE', #15351 ) ;
#14737=DIRECTION ( 'NONE',  ( 1.000000000000000000, -2.891205793294679312E-16, 0.000000000000000000 ) ) ;
#14767=EDGE_CURVE ( 'NONE', #7666, #12252, #12395, .T. ) ;
#14768=EDGE_LOOP ( 'NONE', ( #15153, #15291, #3217, #17695, #3527, #8385, #7880, #3462 ) ) ;
#14783=DIRECTION ( 'NONE',  ( -0.000000000000000000, -0.000000000000000000, -1.000000000000000000 ) ) ;
#14794=VECTOR ( 'NONE', #11294, 1000.000000000000000 ) ;
#14834=AXIS2_PLACEMENT_3D ( 'NONE', #17357, #7341, #13056 ) ;
#14846=VERTEX_POINT ( 'NONE', #2522 ) ;
#14850=ORIENTED_EDGE ( 'NONE', *, *, #3648, .T. ) ;
#14854=DIRECTION ( 'NONE',  ( 0.000000000000000000, -0.000000000000000000, 1.000000000000000000 ) ) ;
#14861=CIRCLE ( 'NONE', #6636, 5.000000000000000000 ) ;
#14915=CARTESIAN_POINT ( 'NONE',  ( -30.00000000000000355, -12.50000000000000178, 0.000000000000000000 ) ) ;
#14918=CARTESIAN_POINT ( 'NONE',  ( 20.00000000000000711, -39.99999999999999289, 3.000000000000000000 ) ) ;
#15012=LINE ( 'NONE', #14918, #460 ) ;
#15016=DIRECTION ( 'NONE',  ( 0.8320502943378440541, -0.5547001962252284812, 0.000000000000000000 ) ) ;
#15032=ORIENTED_EDGE ( 'NONE', *, *, #7806, .F. ) ;
#15087=DIRECTION ( 'NONE',  ( 0.000000000000000000, -1.000000000000000000, 0.000000000000000000 ) ) ;
#15102=CIRCLE ( 'NONE', #1668, 5.000000000000000888 ) ;
#15118=AXIS2_PLACEMENT_3D ( 'NONE', #16949, #9498, #14079 ) ;
#15153=ORIENTED_EDGE ( 'NONE', *, *, #12977, .F. ) ;
#15222=EDGE_CURVE ( 'NONE', #5564, #1182, #6639, .T. ) ;
#15265=EDGE_CURVE ( 'NONE', #8358, #12958, #8538, .T. ) ;
#15291=ORIENTED_EDGE ( 'NONE', *, *, #1186, .T. ) ;
#15292=CARTESIAN_POINT ( 'NONE',  ( -194.9999999999999716, -25.00000000000003197, 3.000000000000000000 ) ) ;
#15303=CIRCLE ( 'NONE', #4626, 2.499999999999995115 ) ;
#15309=DIRECTION ( 'NONE',  ( 1.000000000000000000, 0.000000000000000000, -0.000000000000000000 ) ) ;
#15312=CYLINDRICAL_SURFACE ( 'NONE', #16411, 1.000000000000000000 ) ;
#15324=CARTESIAN_POINT ( 'NONE',  ( -31.48433267924924550, 17.77350098112614418, 0.000000000000000000 ) ) ;
#15351=CARTESIAN_POINT ( 'NONE',  ( 15.00000000000000711, -14.99999999999999645, 3.000000000000000000 ) ) ;
#15354=ORIENTED_EDGE ( 'NONE', *, *, #14626, .T. ) ;
#15357=ORIENTED_EDGE ( 'NONE', *, *, #18112, .F. ) ;
#15362=ADVANCED_FACE ( 'NONE', ( #7598 ), #10063, .F. ) ;
#15368=EDGE_CURVE ( 'NONE', #6155, #14346, #2651, .T. ) ;
#15371=CYLINDRICAL_SURFACE ( 'NONE', #2061, 1.000000000000000000 ) ;
#15405=CARTESIAN_POINT ( 'NONE',  ( -5.999999999999998224, 20.00000000000000000, 3.000000000000000000 ) ) ;
#15408=ORIENTED_EDGE ( 'NONE', *, *, #1544, .T. ) ;
#15427=ADVANCED_FACE ( 'NONE', ( #11882, #26 ), #5844, .T. ) ;
#15447=VECTOR ( 'NONE', #16695, 1000.000000000000000 ) ;
#15527=EDGE_CURVE ( 'NONE', #16287, #13667, #16480, .T. ) ;
#15551=EDGE_CURVE ( 'NONE', #14405, #17750, #17011, .T. ) ;
#15565=ORIENTED_EDGE ( 'NONE', *, *, #13893, .T. ) ;
#15602=CARTESIAN_POINT ( 'NONE',  ( -32.49999999999999289, -12.50000000000000178, 3.000000000000000000 ) ) ;
#15614=CARTESIAN_POINT ( 'NONE',  ( -194.9999999999999716, -45.00000000000003553, 0.000000000000000000 ) ) ;
#15616=CARTESIAN_POINT ( 'NONE',  ( -5.000000000000000888, 17.00000000000000000, 7.000000000000000000 ) ) ;
#15629=DIRECTION ( 'NONE',  ( -0.000000000000000000, -1.000000000000000000, -0.000000000000000000 ) ) ;
#15642=DIRECTION ( 'NONE',  ( -1.000000000000000000, -1.601283208593975514E-16, 0.000000000000000000 ) ) ;
#15716=CARTESIAN_POINT ( 'NONE',  ( 0.000000000000000000, 0.000000000000000000, 0.000000000000000000 ) ) ;
#15718=DIRECTION ( 'NONE',  ( -1.000000000000000000, 0.000000000000000000, 0.000000000000000000 ) ) ;
#15734=CYLINDRICAL_SURFACE ( 'NONE', #13878, 5.000000000000004441 ) ;
#15747=DIRECTION ( 'NONE',  ( 1.000000000000000000, 0.000000000000000000, 0.000000000000000000 ) ) ;
#15750=ORIENTED_EDGE ( 'NONE', *, *, #1186, .F. ) ;
#15764=LINE ( 'NONE', #5448, #14794 ) ;
#15783=AXIS2_PLACEMENT_3D ( 'NONE', #10349, #16751, #15309 ) ;
#15800=CARTESIAN_POINT ( 'NONE',  ( 7.000000000000000000, 8.572527594031473190E-16, 8.000000000000000000 ) ) ;
#15814=SURFACE_STYLE_USAGE ( .BOTH. , #1385 ) ;
#15832=DIRECTION ( 'NONE',  ( -0.000000000000000000, -0.000000000000000000, 1.000000000000000000 ) ) ;
#15911=AXIS2_PLACEMENT_3D ( 'NONE', #4119, #6803, #4021 ) ;
#15923=CARTESIAN_POINT ( 'NONE',  ( -32.49999999999999289, -12.50000000000000178, 3.000000000000000000 ) ) ;
#15925=CARTESIAN_POINT ( 'NONE',  ( 0.000000000000000000, 0.000000000000000000, 8.000000000000000000 ) ) ;
#15930=AXIS2_PLACEMENT_3D ( 'NONE', #11768, #6225, #4509 ) ;
#15937=VERTEX_POINT ( 'NONE', #6221 ) ;
#15954=CARTESIAN_POINT ( 'NONE',  ( 0.000000000000000000, 0.000000000000000000, 0.000000000000000000 ) ) ;
#15974=ORIENTED_EDGE ( 'NONE', *, *, #13893, .F. ) ;
#15997=EDGE_CURVE ( 'NONE', #17750, #12252, #862, .T. ) ;
#16024=EDGE_CURVE ( 'NONE', #10648, #18779, #6979, .T. ) ;
#16029=LINE ( 'NONE', #4374, #4612 ) ;
#16047=VECTOR ( 'NONE', #18149, 1000.000000000000000 ) ;
#16065=PRODUCT_DEFINITION_SHAPE ( 'NONE', 'NONE',  #11634 ) ;
#16086=DIRECTION ( 'NONE',  ( -1.000000000000000000, 1.040834085586084059E-15, 0.000000000000000000 ) ) ;
#16093=AXIS2_PLACEMENT_3D ( 'NONE', #9012, #4421, #10445 ) ;
#16104=CARTESIAN_POINT ( 'NONE',  ( 0.000000000000000000, 0.000000000000000000, 8.000000000000000000 ) ) ;
#16153=ORIENTED_EDGE ( 'NONE', *, *, #10957, .T. ) ;
#16158=CARTESIAN_POINT ( 'NONE',  ( 0.000000000000000000, 0.000000000000000000, 3.000000000000000000 ) ) ;
#16159=ORIENTED_EDGE ( 'NONE', *, *, #1160, .T. ) ;
#16169=PLANE ( 'NONE',  #9739 ) ;
#16218=EDGE_LOOP ( 'NONE', ( #9374, #17105, #11514, #4910 ) ) ;
#16221=CIRCLE ( 'NONE', #4323, 5.000000000000000888 ) ;
#16237=VERTEX_POINT ( 'NONE', #15800 ) ;
#16283=EDGE_CURVE ( 'NONE', #6964, #5564, #17723, .T. ) ;
#16287=VERTEX_POINT ( 'NONE', #13312 ) ;
#16315=ORIENTED_EDGE ( 'NONE', *, *, #12668, .F. ) ;
#16323=VECTOR ( 'NONE', #13403, 1000.000000000000000 ) ;
#16336=EDGE_LOOP ( 'NONE', ( #10087, #2118, #8851, #7793, #8291, #8915, #4451, #15974, #16359, #5135, #6982 ) ) ;
#16351=CARTESIAN_POINT ( 'NONE',  ( -194.9999999999999716, -30.00000000000003197, 0.000000000000000000 ) ) ;
#16353=CIRCLE ( 'NONE', #12065, 5.000000000000000000 ) ;
#16359=ORIENTED_EDGE ( 'NONE', *, *, #15368, .T. ) ;
#16377=VECTOR ( 'NONE', #14111, 1000.000000000000000 ) ;
#16382=EDGE_LOOP ( 'NONE', ( #6083, #276, #8203, #10745 ) ) ;
#16411=AXIS2_PLACEMENT_3D ( 'NONE', #9400, #3368, #18281 ) ;
#16418=ORIENTED_EDGE ( 'NONE', *, *, #586, .T. ) ;
#16455=VERTEX_POINT ( 'NONE', #11026 ) ;
#16478=CARTESIAN_POINT ( 'NONE',  ( -30.00000000000000711, 20.00000000000000000, 3.000000000000000000 ) ) ;
#16480=LINE ( 'NONE', #12078, #4198 ) ;
#16491=FACE_OUTER_BOUND ( 'NONE', #17161, .T. ) ;
#16503=ADVANCED_FACE ( 'NONE', ( #9300 ), #15312, .T. ) ;
#16506=ORIENTED_EDGE ( 'NONE', *, *, #221, .F. ) ;
#16532=EDGE_CURVE ( 'NONE', #16605, #369, #1440, .T. ) ;
#16555=VERTEX_POINT ( 'NONE', #15405 ) ;
#16567=CARTESIAN_POINT ( 'NONE',  ( 15.00000000000000711, -39.99999999999999289, 0.000000000000000000 ) ) ;
#16572=CARTESIAN_POINT ( 'NONE',  ( -199.9999999999999716, -30.00000000000003197, 0.000000000000000000 ) ) ;
#16585=DIRECTION ( 'NONE',  ( -0.000000000000000000, -0.000000000000000000, 1.000000000000000000 ) ) ;
#16586=VECTOR ( 'NONE', #17153, 1000.000000000000000 ) ;
#16596=ORIENTED_EDGE ( 'NONE', *, *, #5786, .F. ) ;
#16605=VERTEX_POINT ( 'NONE', #16991 ) ;
#16615=ORIENTED_EDGE ( 'NONE', *, *, #14312, .F. ) ;
#16647=CARTESIAN_POINT ( 'NONE',  ( -6.000000000000000000, 20.00000000000000000, 4.000000000000000000 ) ) ;
#16650=AXIS2_PLACEMENT_3D ( 'NONE', #162, #8944, #10288 ) ;
#16656=CARTESIAN_POINT ( 'NONE',  ( 20.00000000000000711, -45.00000000000000000, 3.000000000000000000 ) ) ;
#16658=DIRECTION ( 'NONE',  ( -0.000000000000000000, -1.000000000000000000, -0.000000000000000000 ) ) ;
#16692=VERTEX_POINT ( 'NONE', #9313 ) ;
#16695=DIRECTION ( 'NONE',  ( 0.000000000000000000, 0.000000000000000000, -1.000000000000000000 ) ) ;
#16704=CARTESIAN_POINT ( 'NONE',  ( -5.000000000000000000, 0.000000000000000000, 0.000000000000000000 ) ) ;
#16720=LINE ( 'NONE', #3620, #9143 ) ;
#16726=FACE_OUTER_BOUND ( 'NONE', #18348, .T. ) ;
#16731=ORIENTED_EDGE ( 'NONE', *, *, #10831, .T. ) ;
#16751=DIRECTION ( 'NONE',  ( 0.000000000000000000, 0.000000000000000000, 1.000000000000000000 ) ) ;
#16776=CARTESIAN_POINT ( 'NONE',  ( 20.00000000000000711, -45.00000000000000000, 0.000000000000000000 ) ) ;
#16830=DIRECTION ( 'NONE',  ( 0.000000000000000000, -1.000000000000000000, 0.000000000000000000 ) ) ;
#16881=ORIENTED_EDGE ( 'NONE', *, *, #3438, .T. ) ;
#16885=VERTEX_POINT ( 'NONE', #2962 ) ;
#16890=DIRECTION ( 'NONE',  ( -0.000000000000000000, -0.000000000000000000, -1.000000000000000000 ) ) ;
#16904=DIRECTION ( 'NONE',  ( -0.000000000000000000, -0.000000000000000000, -1.000000000000000000 ) ) ;
#16906=CARTESIAN_POINT ( 'NONE',  ( 19.99999999999999645, 15.00000000000000000, 0.000000000000000000 ) ) ;
#16930=VECTOR ( 'NONE', #18881, 1000.000000000000000 ) ;
#16931=DIRECTION ( 'NONE',  ( 1.000000000000000000, 0.000000000000000000, 0.000000000000000000 ) ) ;
#16932=CARTESIAN_POINT ( 'NONE',  ( 15.00000000000000711, -15.99999999999999645, 8.000000000000000000 ) ) ;
#16949=CARTESIAN_POINT ( 'NONE',  ( -194.9999999999999716, -40.00000000000003553, 0.000000000000000000 ) ) ;
#16970=CARTESIAN_POINT ( 'NONE',  ( -199.9999999999999716, -30.00000000000003197, 3.000000000000000000 ) ) ;
#16991=CARTESIAN_POINT ( 'NONE',  ( -5.000000000000000000, 20.00000000000000000, 7.000000000000000000 ) ) ;
#17004=CARTESIAN_POINT ( 'NONE',  ( 19.99999999999999645, 20.00000000000000000, 3.000000000000000000 ) ) ;
#17006=CARTESIAN_POINT ( 'NONE',  ( -4.000000000000000888, 17.00000000000000000, 8.000000000000000000 ) ) ;
#17008=AXIS2_PLACEMENT_3D ( 'NONE', #13025, #1368, #28 ) ;
#17011=CIRCLE ( 'NONE', #13662, 1.000000000000000000 ) ;
#17027=FACE_OUTER_BOUND ( 'NONE', #17566, .T. ) ;
#17030=FACE_BOUND ( 'NONE', #7101, .T. ) ;
#17037=LINE ( 'NONE', #18643, #9353 ) ;
#17065=FILL_AREA_STYLE ('',( #8369 ) ) ;
#17095=DIRECTION ( 'NONE',  ( 0.000000000000000000, 0.000000000000000000, 1.000000000000000000 ) ) ;
#17105=ORIENTED_EDGE ( 'NONE', *, *, #12795, .F. ) ;
#17124=EDGE_CURVE ( 'NONE', #16555, #7666, #1221, .T. ) ;
#17125=DIRECTION ( 'NONE',  ( 1.000000000000000000, -0.000000000000000000, -0.000000000000000000 ) ) ;
#17152=CARTESIAN_POINT ( 'NONE',  ( 0.000000000000000000, 0.000000000000000000, 8.000000000000000000 ) ) ;
#17153=DIRECTION ( 'NONE',  ( -1.000000000000000000, -1.734723475976807094E-16, 0.000000000000000000 ) ) ;
#17161=EDGE_LOOP ( 'NONE', ( #18138, #3067, #13953, #17516 ) ) ;
#17167=LINE ( 'NONE', #15923, #10888 ) ;
#17170=FACE_OUTER_BOUND ( 'NONE', #14255, .T. ) ;
#17200=CARTESIAN_POINT ( 'NONE',  ( 0.000000000000000000, 0.000000000000000000, 8.000000000000000000 ) ) ;
#17205=PLANE ( 'NONE',  #15911 ) ;
#17245=CIRCLE ( 'NONE', #15118, 5.000000000000004441 ) ;
#17249=DIRECTION ( 'NONE',  ( 1.000000000000000000, 0.000000000000000000, 0.000000000000000000 ) ) ;
#17260=FACE_BOUND ( 'NONE', #4788, .T. ) ;
#17288=FACE_OUTER_BOUND ( 'NONE', #839, .T. ) ;
#17293=AXIS2_PLACEMENT_3D ( 'NONE', #12509, #6873, #14228 ) ;
#17313=DIRECTION ( 'NONE',  ( -1.000000000000000000, -2.891205793294679312E-16, 0.000000000000000000 ) ) ;
#17317=ORIENTED_EDGE ( 'NONE', *, *, #12708, .F. ) ;
#17324=DIRECTION ( 'NONE',  ( -0.000000000000000000, -0.000000000000000000, -1.000000000000000000 ) ) ;
#17336=ORIENTED_EDGE ( 'NONE', *, *, #10454, .F. ) ;
#17338=VECTOR ( 'NONE', #7595, 1000.000000000000000 ) ;
#17347=ORIENTED_EDGE ( 'NONE', *, *, #6973, .F. ) ;
#17357=CARTESIAN_POINT ( 'NONE',  ( -4.000000000000006217, 1.156482317317873500E-15, 7.000000000000000000 ) ) ;
#17376=ORIENTED_EDGE ( 'NONE', *, *, #12072, .F. ) ;
#17393=ORIENTED_EDGE ( 'NONE', *, *, #6525, .T. ) ;
#17459=CYLINDRICAL_SURFACE ( 'NONE', #8098, 1.000000000000000000 ) ;
#17471=VERTEX_POINT ( 'NONE', #10588 ) ;
#17491=DIRECTION ( 'NONE',  ( -1.000000000000000000, 0.000000000000000000, 0.000000000000000000 ) ) ;
#17492=ORIENTED_EDGE ( 'NONE', *, *, #1160, .F. ) ;
#17516=ORIENTED_EDGE ( 'NONE', *, *, #13472, .T. ) ;
#17566=EDGE_LOOP ( 'NONE', ( #14703, #18573, #8889, #17920, #3889, #5982, #15565, #6916, #12267, #7791, #14480, #9398 ) ) ;
#17598=DIRECTION ( 'NONE',  ( 2.891205793294679312E-16, -1.000000000000000000, -0.000000000000000000 ) ) ;
#17642=CARTESIAN_POINT ( 'NONE',  ( -30.00000000000000711, 20.00000000000000000, 0.000000000000000000 ) ) ;
#17695=ORIENTED_EDGE ( 'NONE', *, *, #15551, .T. ) ;
#17705=STYLED_ITEM ( 'NONE', ( #18196 ), #3589 ) ;
#17707=LINE ( 'NONE', #7477, #14474 ) ;
#17720=CARTESIAN_POINT ( 'NONE',  ( -5.000000000000000000, 20.00000000000000000, 8.000000000000000000 ) ) ;
#17721=ORIENTED_EDGE ( 'NONE', *, *, #1241, .T. ) ;
#17723=LINE ( 'NONE', #3268, #6325 ) ;
#17750=VERTEX_POINT ( 'NONE', #15616 ) ;
#17769=EDGE_CURVE ( 'NONE', #12252, #6964, #3517, .T. ) ;
#17786=CARTESIAN_POINT ( 'NONE',  ( 15.00000000000000711, -19.99999999999999645, 3.000000000000000000 ) ) ;
#17813=DIRECTION ( 'NONE',  ( -0.000000000000000000, -0.000000000000000000, -1.000000000000000000 ) ) ;
#17822=CARTESIAN_POINT ( 'NONE',  ( -30.00000000000000355, -12.50000000000000178, 3.000000000000000000 ) ) ;
#17826=( LENGTH_UNIT ( ) NAMED_UNIT ( * ) SI_UNIT ( .MILLI., .METRE. ) );
#17840=ORIENTED_EDGE ( 'NONE', *, *, #6489, .T. ) ;
#17859=VECTOR ( 'NONE', #16890, 1000.000000000000000 ) ;
#17866=CIRCLE ( 'NONE', #9608, 7.000000000000000000 ) ;
#17892=ORIENTED_EDGE ( 'NONE', *, *, #16283, .F. ) ;
#17920=ORIENTED_EDGE ( 'NONE', *, *, #8809, .T. ) ;
#17926=CARTESIAN_POINT ( 'NONE',  ( -5.000000000000000000, 20.00000000000000000, 7.000000000000000000 ) ) ;
#17929=DIRECTION ( 'NONE',  ( -1.000000000000000000, -0.000000000000000000, -0.000000000000000000 ) ) ;
#17939=AXIS2_PLACEMENT_3D ( 'NONE', #13787, #2224, #2142 ) ;
#17998=VECTOR ( 'NONE', #17125, 1000.000000000000000 ) ;
#18003=DIRECTION ( 'NONE',  ( 0.000000000000000000, 0.000000000000000000, 1.000000000000000000 ) ) ;
#18009=ADVANCED_FACE ( 'NONE', ( #17027 ), #1870, .F. ) ;
#18057=DIRECTION ( 'NONE',  ( -0.5547001962252284812, -0.8320502943378440541, 0.000000000000000000 ) ) ;
#18071=EDGE_CURVE ( 'NONE', #570, #11716, #963, .T. ) ;
#18077=EDGE_CURVE ( 'NONE', #17471, #13361, #12956, .T. ) ;
#18087=CIRCLE ( 'NONE', #8317, 7.000000000000000000 ) ;
#18112=EDGE_CURVE ( 'NONE', #13667, #11517, #12663, .T. ) ;
#18138=ORIENTED_EDGE ( 'NONE', *, *, #14626, .F. ) ;
#18149=DIRECTION ( 'NONE',  ( -1.000000000000000000, 0.000000000000000000, 0.000000000000000000 ) ) ;
#18162=VECTOR ( 'NONE', #6798, 1000.000000000000000 ) ;
#18179=EDGE_CURVE ( 'NONE', #13361, #2604, #15764, .T. ) ;
#18187=VERTEX_POINT ( 'NONE', #12897 ) ;
#18193=DIRECTION ( 'NONE',  ( 0.000000000000000000, -0.000000000000000000, -1.000000000000000000 ) ) ;
#18196=PRESENTATION_STYLE_ASSIGNMENT (( #7704 ) ) ;
#18225=VECTOR ( 'NONE', #12647, 1000.000000000000000 ) ;
#18228=DIRECTION ( 'NONE',  ( 0.000000000000000000, 0.000000000000000000, 1.000000000000000000 ) ) ;
#18230=CARTESIAN_POINT ( 'NONE',  ( -5.000000000000000888, 17.00000000000000000, 4.000000000000000000 ) ) ;
#18251=DIRECTION ( 'NONE',  ( 0.000000000000000000, 0.000000000000000000, -1.000000000000000000 ) ) ;
#18252=FACE_OUTER_BOUND ( 'NONE', #2669, .T. ) ;
#18281=DIRECTION ( 'NONE',  ( 1.000000000000000000, 2.891205793294679805E-16, 0.000000000000000000 ) ) ;
#18289=ADVANCED_FACE ( 'NONE', ( #7757 ), #1721, .F. ) ;
#18312=EDGE_CURVE ( 'NONE', #6301, #10648, #7809, .T. ) ;
#18318=EDGE_LOOP ( 'NONE', ( #12080, #7985, #6673, #10090, #11911, #4628 ) ) ;
#18348=EDGE_LOOP ( 'NONE', ( #3600, #17376, #11028, #8681 ) ) ;
#18362=FACE_OUTER_BOUND ( 'NONE', #16336, .T. ) ;
#18369=ORIENTED_EDGE ( 'NONE', *, *, #17124, .F. ) ;
#18376=AXIS2_PLACEMENT_3D ( 'NONE', #14915, #13103, #8802 ) ;
#18384=CARTESIAN_POINT ( 'NONE',  ( -5.000000000000000888, 17.00000000000000000, 4.000000000000000000 ) ) ;
#18397=CYLINDRICAL_SURFACE ( 'NONE', #4764, 7.000000000000000000 ) ;
#18421=CARTESIAN_POINT ( 'NONE',  ( -30.00000000000000355, -12.50000000000000178, 3.000000000000000000 ) ) ;
#18430=VECTOR ( 'NONE', #14783, 1000.000000000000000 ) ;
#18459=AXIS2_PLACEMENT_3D ( 'NONE', #16351, #6122, #3232 ) ;
#18464=ADVANCED_FACE ( 'NONE', ( #3627 ), #14036, .F. ) ;
#18519=AXIS2_PLACEMENT_3D ( 'NONE', #3149, #15016, #4801 ) ;
#18527=DIRECTION ( 'NONE',  ( 1.000000000000000000, 0.000000000000000000, 0.000000000000000000 ) ) ;
#18530=AXIS2_PLACEMENT_3D ( 'NONE', #17720, #14737, #8909 ) ;
#18531=ADVANCED_FACE ( 'NONE', ( #761 ), #3532, .T. ) ;
#18545=EDGE_CURVE ( 'NONE', #16692, #7133, #1077, .T. ) ;
#18546=DIRECTION ( 'NONE',  ( 0.000000000000000000, 1.000000000000000000, -0.000000000000000000 ) ) ;
#18551=VECTOR ( 'NONE', #13043, 1000.000000000000000 ) ;
#18554=ORIENTED_EDGE ( 'NONE', *, *, #12749, .F. ) ;
#18573=ORIENTED_EDGE ( 'NONE', *, *, #10115, .T. ) ;
#18623=EDGE_LOOP ( 'NONE', ( #16731, #2458 ) ) ;
#18627=CARTESIAN_POINT ( 'NONE',  ( 12.00000000000000711, -19.99999999999999645, 8.000000000000000000 ) ) ;
#18631=CARTESIAN_POINT ( 'NONE',  ( 15.00000000000000711, -19.99999999999999645, 8.000000000000000000 ) ) ;
#18643=CARTESIAN_POINT ( 'NONE',  ( 7.000000000000000000, 8.572527594031473190E-16, 8.000000000000000000 ) ) ;
#18651=EDGE_LOOP ( 'NONE', ( #9903, #7312, #13658, #4121 ) ) ;
#18673=DIRECTION ( 'NONE',  ( -1.000000000000000000, 0.000000000000000000, 0.000000000000000000 ) ) ;
#18760=ORIENTED_EDGE ( 'NONE', *, *, #12749, .T. ) ;
#18761=VECTOR ( 'NONE', #18057, 1000.000000000000000 ) ;
#18771=CARTESIAN_POINT ( 'NONE',  ( -6.000000000000000888, 17.00000000000000000, 4.000000000000000000 ) ) ;
#18779=VERTEX_POINT ( 'NONE', #5220 ) ;
#18817=AXIS2_PLACEMENT_3D ( 'NONE', #1356, #14271, #9852 ) ;
#18838=VERTEX_POINT ( 'NONE', #10691 ) ;
#18845=CYLINDRICAL_SURFACE ( 'NONE', #18817, 5.000000000000000000 ) ;
#18852=LINE ( 'NONE', #9773, #1654 ) ;
#18876=ORIENTED_EDGE ( 'NONE', *, *, #13489, .T. ) ;
#18881=DIRECTION ( 'NONE',  ( -0.000000000000000000, -0.000000000000000000, 1.000000000000000000 ) ) ;
#18885=FACE_OUTER_BOUND ( 'NONE', #745, .T. ) ;
ENDSEC;
END-ISO-10303-21;
